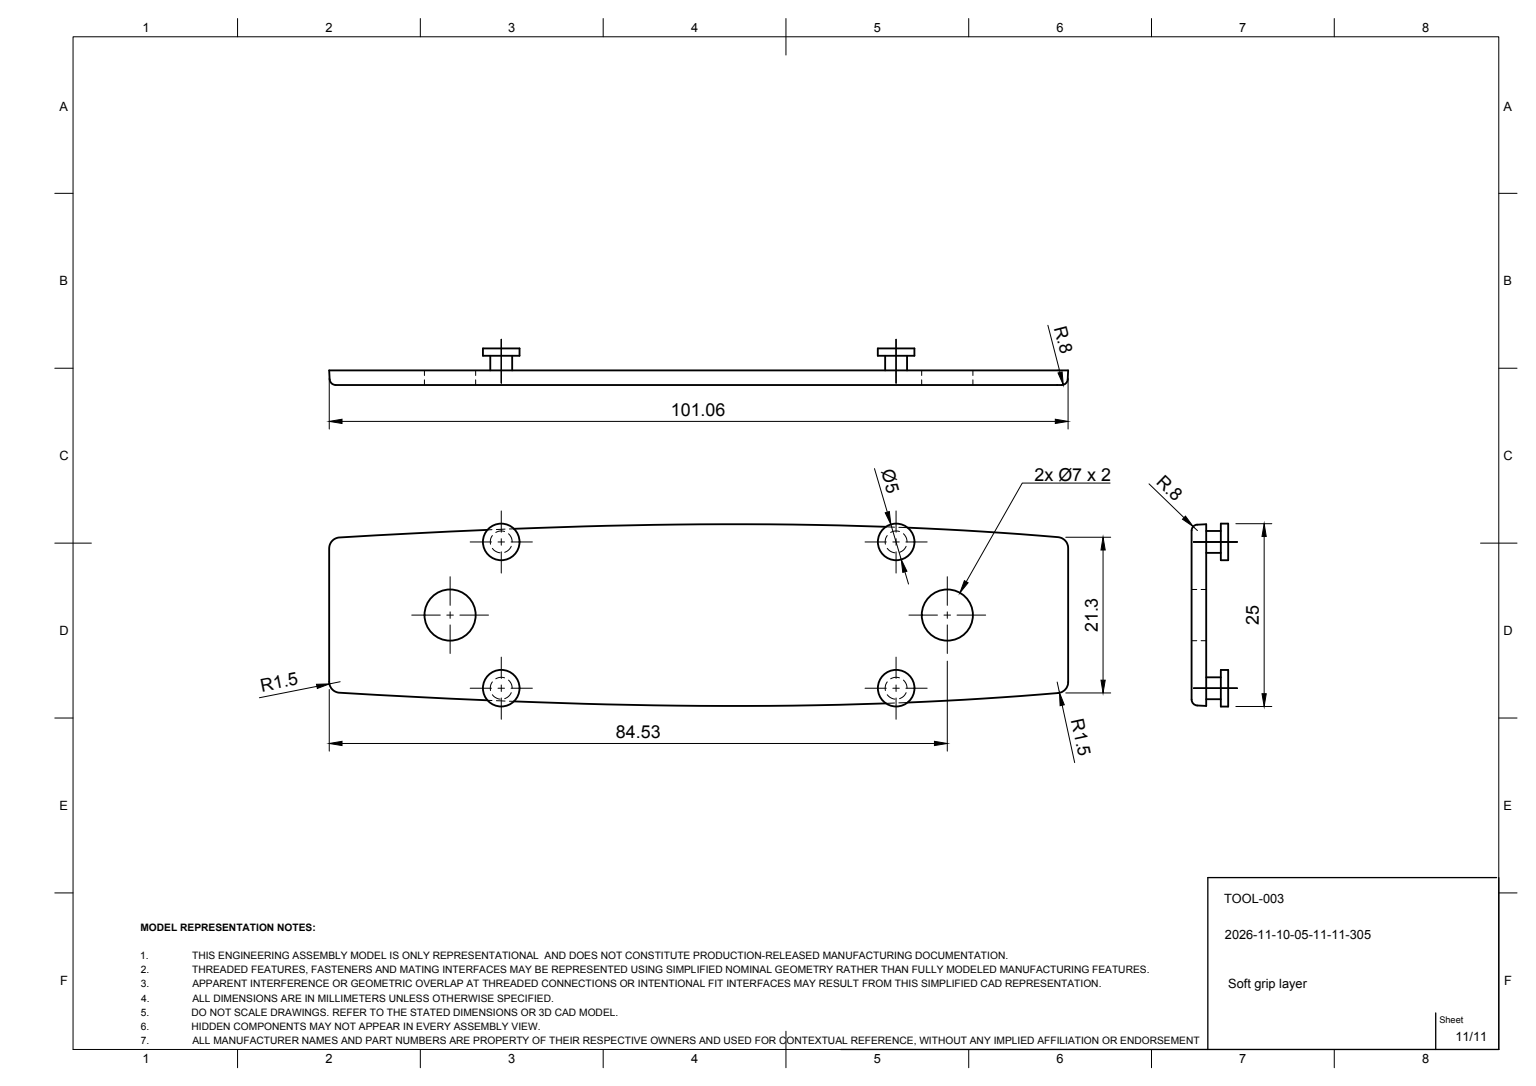
ISO-10303-21;
HEADER;
/* Generated by software containing ST-Developer
 * from STEP Tools, Inc. (www.steptools.com) 
 */

FILE_DESCRIPTION(
/* description */ (''),
/* implementation_level */ '2;1');

FILE_NAME(
/* name */ 'Soft grip layer.step',
/* time_stamp */ '2026-11-10T05:20:16-08:00',
/* author */ (''),
/* organization */ (''),
/* preprocessor_version */ 'ST-DEVELOPER v20.2',
/* originating_system */ 'Autodesk Translation Framework v15.17.0.0',
/* authorisation */ '');

FILE_SCHEMA (('AUTOMOTIVE_DESIGN { 1 0 10303 214 3 1 1 }'));
ENDSEC;

DATA;
#10=MECHANICAL_DESIGN_GEOMETRIC_PRESENTATION_REPRESENTATION('',(#120),#24809);
#100=SHAPE_REPRESENTATION_RELATIONSHIP('SRR','None',#24864,#110);
#110=ADVANCED_BREP_SHAPE_REPRESENTATION('',(#130),#24807);
#120=STYLED_ITEM('',(#24924),#130);
#130=MANIFOLD_SOLID_BREP('Body1',#9897);
#185=FACE_BOUND('',#2432,.T.);
#186=FACE_BOUND('',#2436,.T.);
#187=FACE_BOUND('',#2440,.T.);
#188=FACE_BOUND('',#2444,.T.);
#189=FACE_BOUND('',#2464,.T.);
#190=FACE_BOUND('',#2465,.T.);
#191=FACE_BOUND('',#2470,.T.);
#192=FACE_BOUND('',#2471,.T.);
#193=FACE_BOUND('',#2472,.T.);
#194=FACE_BOUND('',#2473,.T.);
#195=FACE_BOUND('',#2474,.T.);
#196=FACE_BOUND('',#2475,.T.);
#273=B_SPLINE_SURFACE_WITH_KNOTS('',3,3,((#24235,#24236,#24237,#24238,#24239),
(#24240,#24241,#24242,#24243,#24244),(#24245,#24246,#24247,#24248,#24249),
(#24250,#24251,#24252,#24253,#24254),(#24255,#24256,#24257,#24258,#24259)),
 .UNSPECIFIED.,.F.,.F.,.F.,(4,1,4),(4,1,4),(0.,0.571428571428571,1.),(0.,
0.0453052401185593,0.105712226943305),.UNSPECIFIED.);
#274=B_SPLINE_SURFACE_WITH_KNOTS('',3,3,((#24282,#24283,#24284,#24285,#24286),
(#24287,#24288,#24289,#24290,#24291),(#24292,#24293,#24294,#24295,#24296),
(#24297,#24298,#24299,#24300,#24301),(#24302,#24303,#24304,#24305,#24306)),
 .UNSPECIFIED.,.F.,.F.,.F.,(4,1,4),(4,1,4),(0.,0.571428571428571,1.),(0.,
0.0453052401439183,0.105712227002476),.UNSPECIFIED.);
#275=B_SPLINE_SURFACE_WITH_KNOTS('',3,3,((#24320,#24321,#24322,#24323,#24324),
(#24325,#24326,#24327,#24328,#24329),(#24330,#24331,#24332,#24333,#24334),
(#24335,#24336,#24337,#24338,#24339),(#24340,#24341,#24342,#24343,#24344)),
 .UNSPECIFIED.,.F.,.F.,.F.,(4,1,4),(4,1,4),(0.,0.571428571428571,1.),(0.,
4.20509945658767,9.8118987320379),.UNSPECIFIED.);
#276=B_SPLINE_SURFACE_WITH_KNOTS('',3,3,((#24358,#24359,#24360,#24361,#24362),
(#24363,#24364,#24365,#24366,#24367),(#24368,#24369,#24370,#24371,#24372),
(#24373,#24374,#24375,#24376,#24377),(#24378,#24379,#24380,#24381,#24382)),
 .UNSPECIFIED.,.F.,.F.,.F.,(4,1,4),(4,1,4),(0.,0.571428571428571,1.),(0.,
0.0444882141544403,0.103805833027027),.UNSPECIFIED.);
#277=B_SPLINE_SURFACE_WITH_KNOTS('',3,3,((#24402,#24403,#24404,#24405,#24406),
(#24407,#24408,#24409,#24410,#24411),(#24412,#24413,#24414,#24415,#24416),
(#24417,#24418,#24419,#24420,#24421),(#24422,#24423,#24424,#24425,#24426)),
 .UNSPECIFIED.,.F.,.F.,.F.,(4,1,4),(4,1,4),(0.,0.571428571428571,1.),(2.06005858395869E-18,
0.0444882141931362,0.103805833117318),.UNSPECIFIED.);
#278=B_SPLINE_SURFACE_WITH_KNOTS('',3,3,((#24440,#24441,#24442,#24443,#24444),
(#24445,#24446,#24447,#24448,#24449),(#24450,#24451,#24452,#24453,#24454),
(#24455,#24456,#24457,#24458,#24459),(#24460,#24461,#24462,#24463,#24464)),
 .UNSPECIFIED.,.F.,.F.,.F.,(4,1,4),(4,1,4),(0.,0.571428571428571,1.),(0.,
4.20509909783593,9.81189789495051),.UNSPECIFIED.);
#279=B_SPLINE_SURFACE_WITH_KNOTS('',3,3,((#24487,#24488,#24489,#24490),
(#24491,#24492,#24493,#24494),(#24495,#24496,#24497,#24498),(#24499,#24500,
#24501,#24502),(#24503,#24504,#24505,#24506)),.UNSPECIFIED.,.F.,.F.,.F.,
(4,1,4),(4,4),(0.,0.571428571428571,1.),(-0.00268702576369722,0.125151053668407),
 .UNSPECIFIED.);
#280=B_SPLINE_SURFACE_WITH_KNOTS('',3,3,((#24540,#24541,#24542,#24543),
(#24544,#24545,#24546,#24547),(#24548,#24549,#24550,#24551),(#24552,#24553,
#24554,#24555)),.UNSPECIFIED.,.F.,.F.,.F.,(4,4),(4,4),(0.0135518988075539,
0.986045335056424),(0.,0.622596671418298),.UNSPECIFIED.);
#281=B_SPLINE_SURFACE_WITH_KNOTS('',3,3,((#24565,#24566,#24567,#24568),
(#24569,#24570,#24571,#24572),(#24573,#24574,#24575,#24576),(#24577,#24578,
#24579,#24580),(#24581,#24582,#24583,#24584)),.UNSPECIFIED.,.F.,.F.,.F.,
(4,1,4),(4,4),(0.,0.571428571428571,1.),(-0.00281084541253883,0.124959300034279),
 .UNSPECIFIED.);
#282=B_SPLINE_SURFACE_WITH_KNOTS('',3,3,((#24626,#24627,#24628,#24629),
(#24630,#24631,#24632,#24633),(#24634,#24635,#24636,#24637),(#24638,#24639,
#24640,#24641),(#24642,#24643,#24644,#24645)),.UNSPECIFIED.,.F.,.F.,.F.,
(4,1,4),(4,4),(0.,0.571428571428571,1.),(-0.00261432509268751,0.125151053668407),
 .UNSPECIFIED.);
#283=B_SPLINE_SURFACE_WITH_KNOTS('',3,3,((#24679,#24680,#24681,#24682),
(#24683,#24684,#24685,#24686),(#24687,#24688,#24689,#24690),(#24691,#24692,
#24693,#24694),(#24695,#24696,#24697,#24698)),.UNSPECIFIED.,.F.,.F.,.F.,
(4,1,4),(4,4),(0.,0.571428571428571,1.),(-0.00286362952972032,0.124959300034279),
 .UNSPECIFIED.);
#284=B_SPLINE_SURFACE_WITH_KNOTS('',3,3,((#24737,#24738,#24739,#24740),
(#24741,#24742,#24743,#24744),(#24745,#24746,#24747,#24748),(#24749,#24750,
#24751,#24752)),.UNSPECIFIED.,.F.,.F.,.F.,(4,4),(4,4),(0.0139546649435754,
0.986448101192446),(0.,0.622596671418299),.UNSPECIFIED.);
#973=B_SPLINE_CURVE_WITH_KNOTS('',3,(#24264,#24265,#24266,#24267,#24268),
 .UNSPECIFIED.,.F.,.F.,(4,1,4),(-0.105712226943305,-0.0453052401185593,
0.),.UNSPECIFIED.);
#974=B_SPLINE_CURVE_WITH_KNOTS('',3,(#24271,#24272,#24273,#24274,#24275),
 .UNSPECIFIED.,.F.,.F.,(4,1,4),(0.,0.0453052401185593,0.105712226943305),
 .UNSPECIFIED.);
#975=B_SPLINE_CURVE_WITH_KNOTS('',3,(#24310,#24311,#24312,#24313,#24314),
 .UNSPECIFIED.,.F.,.F.,(4,1,4),(-0.105712227002476,-0.0453052401439183,
0.),.UNSPECIFIED.);
#976=B_SPLINE_CURVE_WITH_KNOTS('',3,(#24315,#24316,#24317,#24318,#24319),
 .UNSPECIFIED.,.F.,.F.,(4,1,4),(0.,0.0453052401439183,0.105712227002476),
 .UNSPECIFIED.);
#977=B_SPLINE_CURVE_WITH_KNOTS('',3,(#24348,#24349,#24350,#24351,#24352),
 .UNSPECIFIED.,.F.,.F.,(4,1,4),(-9.8118987320379,-4.20509945658767,0.),
 .UNSPECIFIED.);
#978=B_SPLINE_CURVE_WITH_KNOTS('',3,(#24353,#24354,#24355,#24356,#24357),
 .UNSPECIFIED.,.F.,.F.,(4,1,4),(0.,4.20509945658767,9.8118987320379),
 .UNSPECIFIED.);
#979=B_SPLINE_CURVE_WITH_KNOTS('',3,(#24386,#24387,#24388,#24389,#24390),
 .UNSPECIFIED.,.F.,.F.,(4,1,4),(-0.103805833027027,-0.0444882141544403,
0.),.UNSPECIFIED.);
#980=B_SPLINE_CURVE_WITH_KNOTS('',3,(#24391,#24392,#24393,#24394,#24395),
 .UNSPECIFIED.,.F.,.F.,(4,1,4),(0.,0.0444882141544403,0.103805833027027),
 .UNSPECIFIED.);
#981=B_SPLINE_CURVE_WITH_KNOTS('',3,(#24430,#24431,#24432,#24433,#24434),
 .UNSPECIFIED.,.F.,.F.,(4,1,4),(-0.103805833117318,-0.0444882141931362,
-2.06005858395869E-18),.UNSPECIFIED.);
#982=B_SPLINE_CURVE_WITH_KNOTS('',3,(#24435,#24436,#24437,#24438,#24439),
 .UNSPECIFIED.,.F.,.F.,(4,1,4),(2.06005858395869E-18,0.0444882141931362,
0.103805833117318),.UNSPECIFIED.);
#983=B_SPLINE_CURVE_WITH_KNOTS('',3,(#24465,#24466,#24467,#24468,#24469),
 .UNSPECIFIED.,.F.,.F.,(4,1,4),(-9.81189789495051,-4.20509909783593,0.),
 .UNSPECIFIED.);
#984=B_SPLINE_CURVE_WITH_KNOTS('',3,(#24470,#24471,#24472,#24473,#24474),
 .UNSPECIFIED.,.F.,.F.,(4,1,4),(0.,4.20509909783593,9.81189789495051),
 .UNSPECIFIED.);
#985=B_SPLINE_CURVE_WITH_KNOTS('',3,(#24477,#24478,#24479,#24480),
 .UNSPECIFIED.,.F.,.F.,(4,4),(0.00062434729305816,0.125151053668407),
 .UNSPECIFIED.);
#986=B_SPLINE_CURVE_WITH_KNOTS('',3,(#24483,#24484,#24485,#24486),
 .UNSPECIFIED.,.F.,.F.,(4,4),(-0.125151053668407,-0.000624347293058304),
 .UNSPECIFIED.);
#987=B_SPLINE_CURVE_WITH_KNOTS('',3,(#24508,#24509,#24510,#24511),
 .UNSPECIFIED.,.F.,.F.,(4,4),(-0.124859357077656,3.91613824701764E-16),
 .UNSPECIFIED.);
#988=B_SPLINE_CURVE_WITH_KNOTS('',3,(#24512,#24513,#24514,#24515,#24516,
#24517,#24518,#24519,#24520,#24521,#24522,#24523,#24524,#24525,#24526,#24527,
#24528,#24529,#24530,#24531,#24532,#24533,#24534,#24535,#24536,#24537,#24538,
#24539),.UNSPECIFIED.,.F.,.F.,(4,3,3,3,3,3,3,3,3,4),(0.,0.0322709922822142,
0.0586131010579366,0.0908535483049993,0.095660418056781,0.117090121226367,
0.14947943031994,0.17008966569926,0.202270498561131,0.223122165115773),
 .UNSPECIFIED.);
#989=B_SPLINE_CURVE_WITH_KNOTS('',3,(#24557,#24558,#24559,#24560),
 .UNSPECIFIED.,.F.,.F.,(4,4),(1.57426155444895E-16,0.124757292074316),
 .UNSPECIFIED.);
#990=B_SPLINE_CURVE_WITH_KNOTS('',3,(#24561,#24562,#24563,#24564),
 .UNSPECIFIED.,.F.,.F.,(4,4),(0.0135518988075539,0.986045335056425),
 .UNSPECIFIED.);
#991=B_SPLINE_CURVE_WITH_KNOTS('',3,(#24586,#24587,#24588,#24589),
 .UNSPECIFIED.,.F.,.F.,(4,4),(-0.124959300034279,-0.000432357919845506),
 .UNSPECIFIED.);
#992=B_SPLINE_CURVE_WITH_KNOTS('',3,(#24590,#24591,#24592,#24593,#24594,
#24595,#24596,#24597,#24598,#24599,#24600,#24601,#24602,#24603,#24604,#24605,
#24606,#24607,#24608,#24609,#24610,#24611,#24612,#24613,#24614,#24615,#24616,
#24617),.UNSPECIFIED.,.F.,.F.,(4,3,3,3,3,3,3,3,3,4),(0.,0.0322720371751271,
0.0586511315716134,0.0908889384397039,0.0974306796249642,0.117149930269381,
0.149553095257184,0.172178760978465,0.204364325027201,0.227238249760569),
 .UNSPECIFIED.);
#993=B_SPLINE_CURVE_WITH_KNOTS('',3,(#24621,#24622,#24623,#24624),
 .UNSPECIFIED.,.F.,.F.,(4,4),(0.000432357919845864,0.124959300034279),
 .UNSPECIFIED.);
#994=B_SPLINE_CURVE_WITH_KNOTS('',3,(#24647,#24648,#24649,#24650,#24651,
#24652,#24653,#24654,#24655,#24656,#24657,#24658,#24659,#24660,#24661,#24662,
#24663,#24664,#24665,#24666,#24667,#24668,#24669,#24670,#24671,#24672,#24673,
#24674),.UNSPECIFIED.,.F.,.F.,(4,3,3,3,3,3,3,3,3,4),(0.,0.0322770007607458,
0.0586509099358757,0.0908890592373506,0.0956758252683957,0.117149647541228,
0.149540928065794,0.17012301918783,0.202296660223156,0.2231241621482),
 .UNSPECIFIED.);
#995=B_SPLINE_CURVE_WITH_KNOTS('',3,(#24675,#24676,#24677,#24678),
 .UNSPECIFIED.,.F.,.F.,(4,4),(1.94722710178397E-16,0.124859357077656),
 .UNSPECIFIED.);
#996=B_SPLINE_CURVE_WITH_KNOTS('',3,(#24700,#24701,#24702,#24703),
 .UNSPECIFIED.,.F.,.F.,(4,4),(-0.124757292074297,-2.43294967505747E-16),
 .UNSPECIFIED.);
#997=B_SPLINE_CURVE_WITH_KNOTS('',3,(#24704,#24705,#24706,#24707,#24708,
#24709,#24710,#24711,#24712,#24713,#24714,#24715,#24716,#24717,#24718,#24719,
#24720,#24721,#24722,#24723,#24724,#24725,#24726,#24727,#24728,#24729,#24730,
#24731),.UNSPECIFIED.,.F.,.F.,(4,3,3,3,3,3,3,3,3,4),(0.,0.0322677829554273,
0.0586251784806003,0.0908644978360146,0.097419835848357,0.117108565494702,
0.149510109206484,0.172155480916619,0.204345933772221,0.227236831322489),
 .UNSPECIFIED.);
#998=B_SPLINE_CURVE_WITH_KNOTS('',3,(#24733,#24734,#24735,#24736),
 .UNSPECIFIED.,.F.,.F.,(4,4),(0.0139546649435756,0.986448101192446),
 .UNSPECIFIED.);
#1296=PLANE('',#10602);
#1297=PLANE('',#10607);
#1298=PLANE('',#10608);
#1299=PLANE('',#10613);
#1300=PLANE('',#10614);
#1301=PLANE('',#10619);
#1302=PLANE('',#10620);
#1303=PLANE('',#10625);
#1304=PLANE('',#10644);
#1305=PLANE('',#10645);
#1306=PLANE('',#10646);
#1307=PLANE('',#10647);
#1823=FACE_OUTER_BOUND('',#2429,.T.);
#1824=FACE_OUTER_BOUND('',#2430,.T.);
#1825=FACE_OUTER_BOUND('',#2431,.T.);
#1826=FACE_OUTER_BOUND('',#2433,.T.);
#1827=FACE_OUTER_BOUND('',#2434,.T.);
#1828=FACE_OUTER_BOUND('',#2435,.T.);
#1829=FACE_OUTER_BOUND('',#2437,.T.);
#1830=FACE_OUTER_BOUND('',#2438,.T.);
#1831=FACE_OUTER_BOUND('',#2439,.T.);
#1832=FACE_OUTER_BOUND('',#2441,.T.);
#1833=FACE_OUTER_BOUND('',#2442,.T.);
#1834=FACE_OUTER_BOUND('',#2443,.T.);
#1835=FACE_OUTER_BOUND('',#2445,.T.);
#1836=FACE_OUTER_BOUND('',#2446,.T.);
#1837=FACE_OUTER_BOUND('',#2447,.T.);
#1838=FACE_OUTER_BOUND('',#2448,.T.);
#1839=FACE_OUTER_BOUND('',#2449,.T.);
#1840=FACE_OUTER_BOUND('',#2450,.T.);
#1841=FACE_OUTER_BOUND('',#2451,.T.);
#1842=FACE_OUTER_BOUND('',#2452,.T.);
#1843=FACE_OUTER_BOUND('',#2453,.T.);
#1844=FACE_OUTER_BOUND('',#2454,.T.);
#1845=FACE_OUTER_BOUND('',#2455,.T.);
#1846=FACE_OUTER_BOUND('',#2456,.T.);
#1847=FACE_OUTER_BOUND('',#2457,.T.);
#1848=FACE_OUTER_BOUND('',#2458,.T.);
#1849=FACE_OUTER_BOUND('',#2459,.T.);
#1850=FACE_OUTER_BOUND('',#2460,.T.);
#1851=FACE_OUTER_BOUND('',#2461,.T.);
#1852=FACE_OUTER_BOUND('',#2462,.T.);
#1853=FACE_OUTER_BOUND('',#2463,.T.);
#1854=FACE_OUTER_BOUND('',#2466,.T.);
#1855=FACE_OUTER_BOUND('',#2467,.T.);
#1856=FACE_OUTER_BOUND('',#2468,.T.);
#1857=FACE_OUTER_BOUND('',#2469,.T.);
#1858=FACE_OUTER_BOUND('',#2476,.T.);
#2429=EDGE_LOOP('',(#9045,#9046,#9047,#9048));
#2430=EDGE_LOOP('',(#9049,#9050,#9051,#9052));
#2431=EDGE_LOOP('',(#9053));
#2432=EDGE_LOOP('',(#9054));
#2433=EDGE_LOOP('',(#9055,#9056,#9057,#9058));
#2434=EDGE_LOOP('',(#9059));
#2435=EDGE_LOOP('',(#9060));
#2436=EDGE_LOOP('',(#9061));
#2437=EDGE_LOOP('',(#9062,#9063,#9064,#9065));
#2438=EDGE_LOOP('',(#9066));
#2439=EDGE_LOOP('',(#9067));
#2440=EDGE_LOOP('',(#9068));
#2441=EDGE_LOOP('',(#9069,#9070,#9071,#9072));
#2442=EDGE_LOOP('',(#9073));
#2443=EDGE_LOOP('',(#9074));
#2444=EDGE_LOOP('',(#9075));
#2445=EDGE_LOOP('',(#9076,#9077,#9078,#9079));
#2446=EDGE_LOOP('',(#9080));
#2447=EDGE_LOOP('',(#9081,#9082,#9083,#9084));
#2448=EDGE_LOOP('',(#9085,#9086,#9087,#9088));
#2449=EDGE_LOOP('',(#9089,#9090,#9091,#9092));
#2450=EDGE_LOOP('',(#9093,#9094,#9095,#9096));
#2451=EDGE_LOOP('',(#9097,#9098,#9099,#9100));
#2452=EDGE_LOOP('',(#9101,#9102,#9103,#9104));
#2453=EDGE_LOOP('',(#9105,#9106,#9107,#9108));
#2454=EDGE_LOOP('',(#9109,#9110,#9111,#9112));
#2455=EDGE_LOOP('',(#9113,#9114,#9115,#9116));
#2456=EDGE_LOOP('',(#9117,#9118,#9119,#9120));
#2457=EDGE_LOOP('',(#9121,#9122,#9123,#9124));
#2458=EDGE_LOOP('',(#9125,#9126,#9127,#9128));
#2459=EDGE_LOOP('',(#9129,#9130,#9131,#9132));
#2460=EDGE_LOOP('',(#9133,#9134,#9135,#9136));
#2461=EDGE_LOOP('',(#9137,#9138,#9139,#9140));
#2462=EDGE_LOOP('',(#9141,#9142,#9143,#9144));
#2463=EDGE_LOOP('',(#9145,#9146,#9147,#9148,#9149,#9150,#9151,#9152));
#2464=EDGE_LOOP('',(#9153));
#2465=EDGE_LOOP('',(#9154));
#2466=EDGE_LOOP('',(#9155,#9156,#9157,#9158));
#2467=EDGE_LOOP('',(#9159,#9160,#9161,#9162));
#2468=EDGE_LOOP('',(#9163,#9164,#9165,#9166));
#2469=EDGE_LOOP('',(#9167,#9168,#9169,#9170,#9171,#9172,#9173,#9174));
#2470=EDGE_LOOP('',(#9175));
#2471=EDGE_LOOP('',(#9176));
#2472=EDGE_LOOP('',(#9177));
#2473=EDGE_LOOP('',(#9178));
#2474=EDGE_LOOP('',(#9179));
#2475=EDGE_LOOP('',(#9180));
#2476=EDGE_LOOP('',(#9181,#9182,#9183,#9184));
#3053=LINE('',#24171,#3641);
#3054=LINE('',#24177,#3642);
#3055=LINE('',#24187,#3643);
#3056=LINE('',#24197,#3644);
#3057=LINE('',#24207,#3645);
#3058=LINE('',#24217,#3646);
#3059=LINE('',#24221,#3647);
#3060=LINE('',#24225,#3648);
#3061=LINE('',#24229,#3649);
#3062=LINE('',#24233,#3650);
#3063=LINE('',#24280,#3651);
#3064=LINE('',#24281,#3652);
#3065=LINE('',#24400,#3653);
#3066=LINE('',#24401,#3654);
#3067=LINE('',#24482,#3655);
#3068=LINE('',#24625,#3656);
#3641=VECTOR('',#12419,0.35);
#3642=VECTOR('',#12426,0.35);
#3643=VECTOR('',#12439,0.25);
#3644=VECTOR('',#12452,0.25);
#3645=VECTOR('',#12465,0.25);
#3646=VECTOR('',#12478,0.25);
#3647=VECTOR('',#12483,0.15);
#3648=VECTOR('',#12488,0.15);
#3649=VECTOR('',#12493,0.15);
#3650=VECTOR('',#12498,0.15);
#3651=VECTOR('',#12509,1.);
#3652=VECTOR('',#12510,1.);
#3653=VECTOR('',#12521,1.);
#3654=VECTOR('',#12522,1.);
#3655=VECTOR('',#12527,1.);
#3656=VECTOR('',#12532,1.);
#3795=CIRCLE('',#10597,0.35);
#3796=CIRCLE('',#10598,0.35);
#3797=CIRCLE('',#10600,0.35);
#3798=CIRCLE('',#10601,0.35);
#3799=CIRCLE('',#10603,0.25);
#3800=CIRCLE('',#10604,0.15);
#3801=CIRCLE('',#10606,0.25);
#3802=CIRCLE('',#10609,0.25);
#3803=CIRCLE('',#10610,0.15);
#3804=CIRCLE('',#10612,0.25);
#3805=CIRCLE('',#10615,0.25);
#3806=CIRCLE('',#10616,0.15);
#3807=CIRCLE('',#10618,0.25);
#3808=CIRCLE('',#10621,0.25);
#3809=CIRCLE('',#10622,0.15);
#3810=CIRCLE('',#10624,0.25);
#3811=CIRCLE('',#10627,0.15);
#3812=CIRCLE('',#10629,0.15);
#3813=CIRCLE('',#10631,0.15);
#3814=CIRCLE('',#10633,0.15);
#3815=CIRCLE('',#10634,0.0800000000000001);
#3816=CIRCLE('',#10635,0.0799999999999999);
#3817=CIRCLE('',#10637,0.0800000000000001);
#3818=CIRCLE('',#10638,0.0800000000000001);
#3819=CIRCLE('',#10639,0.0800000000000001);
#3820=CIRCLE('',#10640,0.0800000000000001);
#3821=CIRCLE('',#10642,0.0800000000000001);
#3822=CIRCLE('',#10643,0.0800000000000001);
#4739=VERTEX_POINT('',#24168);
#4740=VERTEX_POINT('',#24170);
#4741=VERTEX_POINT('',#24174);
#4742=VERTEX_POINT('',#24176);
#4743=VERTEX_POINT('',#24180);
#4744=VERTEX_POINT('',#24182);
#4745=VERTEX_POINT('',#24185);
#4746=VERTEX_POINT('',#24190);
#4747=VERTEX_POINT('',#24192);
#4748=VERTEX_POINT('',#24195);
#4749=VERTEX_POINT('',#24200);
#4750=VERTEX_POINT('',#24202);
#4751=VERTEX_POINT('',#24205);
#4752=VERTEX_POINT('',#24210);
#4753=VERTEX_POINT('',#24212);
#4754=VERTEX_POINT('',#24215);
#4755=VERTEX_POINT('',#24220);
#4756=VERTEX_POINT('',#24224);
#4757=VERTEX_POINT('',#24228);
#4758=VERTEX_POINT('',#24232);
#4759=VERTEX_POINT('',#24260);
#4760=VERTEX_POINT('',#24261);
#4761=VERTEX_POINT('',#24263);
#4762=VERTEX_POINT('',#24269);
#4763=VERTEX_POINT('',#24277);
#4764=VERTEX_POINT('',#24278);
#4765=VERTEX_POINT('',#24307);
#4766=VERTEX_POINT('',#24308);
#4767=VERTEX_POINT('',#24345);
#4768=VERTEX_POINT('',#24346);
#4769=VERTEX_POINT('',#24383);
#4770=VERTEX_POINT('',#24384);
#4771=VERTEX_POINT('',#24397);
#4772=VERTEX_POINT('',#24398);
#4773=VERTEX_POINT('',#24427);
#4774=VERTEX_POINT('',#24428);
#4775=VERTEX_POINT('',#24476);
#4776=VERTEX_POINT('',#24481);
#4777=VERTEX_POINT('',#24507);
#4778=VERTEX_POINT('',#24556);
#4779=VERTEX_POINT('',#24585);
#4780=VERTEX_POINT('',#24620);
#4781=VERTEX_POINT('',#24646);
#4782=VERTEX_POINT('',#24699);
#6181=EDGE_CURVE('',#4739,#4739,#3795,.T.);
#6182=EDGE_CURVE('',#4739,#4740,#3053,.T.);
#6183=EDGE_CURVE('',#4740,#4740,#3796,.T.);
#6184=EDGE_CURVE('',#4741,#4741,#3797,.T.);
#6185=EDGE_CURVE('',#4741,#4742,#3054,.T.);
#6186=EDGE_CURVE('',#4742,#4742,#3798,.T.);
#6187=EDGE_CURVE('',#4743,#4743,#3799,.T.);
#6188=EDGE_CURVE('',#4744,#4744,#3800,.T.);
#6189=EDGE_CURVE('',#4745,#4745,#3801,.T.);
#6190=EDGE_CURVE('',#4745,#4743,#3055,.T.);
#6191=EDGE_CURVE('',#4746,#4746,#3802,.T.);
#6192=EDGE_CURVE('',#4747,#4747,#3803,.T.);
#6193=EDGE_CURVE('',#4748,#4748,#3804,.T.);
#6194=EDGE_CURVE('',#4748,#4746,#3056,.T.);
#6195=EDGE_CURVE('',#4749,#4749,#3805,.T.);
#6196=EDGE_CURVE('',#4750,#4750,#3806,.T.);
#6197=EDGE_CURVE('',#4751,#4751,#3807,.T.);
#6198=EDGE_CURVE('',#4751,#4749,#3057,.T.);
#6199=EDGE_CURVE('',#4752,#4752,#3808,.T.);
#6200=EDGE_CURVE('',#4753,#4753,#3809,.T.);
#6201=EDGE_CURVE('',#4754,#4754,#3810,.T.);
#6202=EDGE_CURVE('',#4754,#4752,#3058,.T.);
#6203=EDGE_CURVE('',#4744,#4755,#3059,.T.);
#6204=EDGE_CURVE('',#4755,#4755,#3811,.T.);
#6205=EDGE_CURVE('',#4747,#4756,#3060,.T.);
#6206=EDGE_CURVE('',#4756,#4756,#3812,.T.);
#6207=EDGE_CURVE('',#4750,#4757,#3061,.T.);
#6208=EDGE_CURVE('',#4757,#4757,#3813,.T.);
#6209=EDGE_CURVE('',#4753,#4758,#3062,.T.);
#6210=EDGE_CURVE('',#4758,#4758,#3814,.T.);
#6211=EDGE_CURVE('',#4759,#4760,#3815,.T.);
#6212=EDGE_CURVE('',#4760,#4761,#973,.T.);
#6213=EDGE_CURVE('',#4761,#4762,#3816,.T.);
#6214=EDGE_CURVE('',#4762,#4759,#974,.T.);
#6215=EDGE_CURVE('',#4763,#4764,#3817,.T.);
#6216=EDGE_CURVE('',#4764,#4760,#3063,.T.);
#6217=EDGE_CURVE('',#4759,#4763,#3064,.T.);
#6218=EDGE_CURVE('',#4765,#4766,#3818,.T.);
#6219=EDGE_CURVE('',#4766,#4764,#975,.T.);
#6220=EDGE_CURVE('',#4763,#4765,#976,.T.);
#6221=EDGE_CURVE('',#4767,#4768,#3819,.T.);
#6222=EDGE_CURVE('',#4768,#4766,#977,.T.);
#6223=EDGE_CURVE('',#4765,#4767,#978,.T.);
#6224=EDGE_CURVE('',#4769,#4770,#3820,.T.);
#6225=EDGE_CURVE('',#4770,#4768,#979,.T.);
#6226=EDGE_CURVE('',#4767,#4769,#980,.T.);
#6227=EDGE_CURVE('',#4771,#4772,#3821,.T.);
#6228=EDGE_CURVE('',#4772,#4770,#3065,.T.);
#6229=EDGE_CURVE('',#4769,#4771,#3066,.T.);
#6230=EDGE_CURVE('',#4773,#4774,#3822,.T.);
#6231=EDGE_CURVE('',#4774,#4772,#981,.T.);
#6232=EDGE_CURVE('',#4771,#4773,#982,.T.);
#6233=EDGE_CURVE('',#4761,#4774,#983,.T.);
#6234=EDGE_CURVE('',#4773,#4762,#984,.T.);
#6235=EDGE_CURVE('',#4775,#4772,#985,.T.);
#6236=EDGE_CURVE('',#4776,#4775,#3067,.T.);
#6237=EDGE_CURVE('',#4770,#4776,#986,.T.);
#6238=EDGE_CURVE('',#4774,#4777,#987,.T.);
#6239=EDGE_CURVE('',#4777,#4775,#988,.T.);
#6240=EDGE_CURVE('',#4778,#4761,#989,.T.);
#6241=EDGE_CURVE('',#4777,#4778,#990,.T.);
#6242=EDGE_CURVE('',#4760,#4779,#991,.T.);
#6243=EDGE_CURVE('',#4779,#4778,#992,.T.);
#6244=EDGE_CURVE('',#4780,#4764,#993,.T.);
#6245=EDGE_CURVE('',#4779,#4780,#3068,.T.);
#6246=EDGE_CURVE('',#4776,#4781,#994,.T.);
#6247=EDGE_CURVE('',#4781,#4768,#995,.T.);
#6248=EDGE_CURVE('',#4766,#4782,#996,.T.);
#6249=EDGE_CURVE('',#4782,#4780,#997,.T.);
#6250=EDGE_CURVE('',#4782,#4781,#998,.T.);
#9045=ORIENTED_EDGE('',*,*,#6181,.F.);
#9046=ORIENTED_EDGE('',*,*,#6182,.T.);
#9047=ORIENTED_EDGE('',*,*,#6183,.F.);
#9048=ORIENTED_EDGE('',*,*,#6182,.F.);
#9049=ORIENTED_EDGE('',*,*,#6184,.F.);
#9050=ORIENTED_EDGE('',*,*,#6185,.T.);
#9051=ORIENTED_EDGE('',*,*,#6186,.F.);
#9052=ORIENTED_EDGE('',*,*,#6185,.F.);
#9053=ORIENTED_EDGE('',*,*,#6187,.T.);
#9054=ORIENTED_EDGE('',*,*,#6188,.T.);
#9055=ORIENTED_EDGE('',*,*,#6189,.F.);
#9056=ORIENTED_EDGE('',*,*,#6190,.T.);
#9057=ORIENTED_EDGE('',*,*,#6187,.F.);
#9058=ORIENTED_EDGE('',*,*,#6190,.F.);
#9059=ORIENTED_EDGE('',*,*,#6189,.T.);
#9060=ORIENTED_EDGE('',*,*,#6191,.T.);
#9061=ORIENTED_EDGE('',*,*,#6192,.T.);
#9062=ORIENTED_EDGE('',*,*,#6193,.F.);
#9063=ORIENTED_EDGE('',*,*,#6194,.T.);
#9064=ORIENTED_EDGE('',*,*,#6191,.F.);
#9065=ORIENTED_EDGE('',*,*,#6194,.F.);
#9066=ORIENTED_EDGE('',*,*,#6193,.T.);
#9067=ORIENTED_EDGE('',*,*,#6195,.T.);
#9068=ORIENTED_EDGE('',*,*,#6196,.T.);
#9069=ORIENTED_EDGE('',*,*,#6197,.F.);
#9070=ORIENTED_EDGE('',*,*,#6198,.T.);
#9071=ORIENTED_EDGE('',*,*,#6195,.F.);
#9072=ORIENTED_EDGE('',*,*,#6198,.F.);
#9073=ORIENTED_EDGE('',*,*,#6197,.T.);
#9074=ORIENTED_EDGE('',*,*,#6199,.T.);
#9075=ORIENTED_EDGE('',*,*,#6200,.T.);
#9076=ORIENTED_EDGE('',*,*,#6201,.F.);
#9077=ORIENTED_EDGE('',*,*,#6202,.T.);
#9078=ORIENTED_EDGE('',*,*,#6199,.F.);
#9079=ORIENTED_EDGE('',*,*,#6202,.F.);
#9080=ORIENTED_EDGE('',*,*,#6201,.T.);
#9081=ORIENTED_EDGE('',*,*,#6188,.F.);
#9082=ORIENTED_EDGE('',*,*,#6203,.T.);
#9083=ORIENTED_EDGE('',*,*,#6204,.F.);
#9084=ORIENTED_EDGE('',*,*,#6203,.F.);
#9085=ORIENTED_EDGE('',*,*,#6192,.F.);
#9086=ORIENTED_EDGE('',*,*,#6205,.T.);
#9087=ORIENTED_EDGE('',*,*,#6206,.F.);
#9088=ORIENTED_EDGE('',*,*,#6205,.F.);
#9089=ORIENTED_EDGE('',*,*,#6196,.F.);
#9090=ORIENTED_EDGE('',*,*,#6207,.T.);
#9091=ORIENTED_EDGE('',*,*,#6208,.F.);
#9092=ORIENTED_EDGE('',*,*,#6207,.F.);
#9093=ORIENTED_EDGE('',*,*,#6200,.F.);
#9094=ORIENTED_EDGE('',*,*,#6209,.T.);
#9095=ORIENTED_EDGE('',*,*,#6210,.F.);
#9096=ORIENTED_EDGE('',*,*,#6209,.F.);
#9097=ORIENTED_EDGE('',*,*,#6211,.T.);
#9098=ORIENTED_EDGE('',*,*,#6212,.T.);
#9099=ORIENTED_EDGE('',*,*,#6213,.T.);
#9100=ORIENTED_EDGE('',*,*,#6214,.T.);
#9101=ORIENTED_EDGE('',*,*,#6215,.T.);
#9102=ORIENTED_EDGE('',*,*,#6216,.T.);
#9103=ORIENTED_EDGE('',*,*,#6211,.F.);
#9104=ORIENTED_EDGE('',*,*,#6217,.T.);
#9105=ORIENTED_EDGE('',*,*,#6218,.T.);
#9106=ORIENTED_EDGE('',*,*,#6219,.T.);
#9107=ORIENTED_EDGE('',*,*,#6215,.F.);
#9108=ORIENTED_EDGE('',*,*,#6220,.T.);
#9109=ORIENTED_EDGE('',*,*,#6221,.T.);
#9110=ORIENTED_EDGE('',*,*,#6222,.T.);
#9111=ORIENTED_EDGE('',*,*,#6218,.F.);
#9112=ORIENTED_EDGE('',*,*,#6223,.T.);
#9113=ORIENTED_EDGE('',*,*,#6224,.T.);
#9114=ORIENTED_EDGE('',*,*,#6225,.T.);
#9115=ORIENTED_EDGE('',*,*,#6221,.F.);
#9116=ORIENTED_EDGE('',*,*,#6226,.T.);
#9117=ORIENTED_EDGE('',*,*,#6227,.T.);
#9118=ORIENTED_EDGE('',*,*,#6228,.T.);
#9119=ORIENTED_EDGE('',*,*,#6224,.F.);
#9120=ORIENTED_EDGE('',*,*,#6229,.T.);
#9121=ORIENTED_EDGE('',*,*,#6230,.T.);
#9122=ORIENTED_EDGE('',*,*,#6231,.T.);
#9123=ORIENTED_EDGE('',*,*,#6227,.F.);
#9124=ORIENTED_EDGE('',*,*,#6232,.T.);
#9125=ORIENTED_EDGE('',*,*,#6213,.F.);
#9126=ORIENTED_EDGE('',*,*,#6233,.T.);
#9127=ORIENTED_EDGE('',*,*,#6230,.F.);
#9128=ORIENTED_EDGE('',*,*,#6234,.T.);
#9129=ORIENTED_EDGE('',*,*,#6228,.F.);
#9130=ORIENTED_EDGE('',*,*,#6235,.F.);
#9131=ORIENTED_EDGE('',*,*,#6236,.F.);
#9132=ORIENTED_EDGE('',*,*,#6237,.F.);
#9133=ORIENTED_EDGE('',*,*,#6231,.F.);
#9134=ORIENTED_EDGE('',*,*,#6238,.T.);
#9135=ORIENTED_EDGE('',*,*,#6239,.T.);
#9136=ORIENTED_EDGE('',*,*,#6235,.T.);
#9137=ORIENTED_EDGE('',*,*,#6233,.F.);
#9138=ORIENTED_EDGE('',*,*,#6240,.F.);
#9139=ORIENTED_EDGE('',*,*,#6241,.F.);
#9140=ORIENTED_EDGE('',*,*,#6238,.F.);
#9141=ORIENTED_EDGE('',*,*,#6212,.F.);
#9142=ORIENTED_EDGE('',*,*,#6242,.T.);
#9143=ORIENTED_EDGE('',*,*,#6243,.T.);
#9144=ORIENTED_EDGE('',*,*,#6240,.T.);
#9145=ORIENTED_EDGE('',*,*,#6214,.F.);
#9146=ORIENTED_EDGE('',*,*,#6234,.F.);
#9147=ORIENTED_EDGE('',*,*,#6232,.F.);
#9148=ORIENTED_EDGE('',*,*,#6229,.F.);
#9149=ORIENTED_EDGE('',*,*,#6226,.F.);
#9150=ORIENTED_EDGE('',*,*,#6223,.F.);
#9151=ORIENTED_EDGE('',*,*,#6220,.F.);
#9152=ORIENTED_EDGE('',*,*,#6217,.F.);
#9153=ORIENTED_EDGE('',*,*,#6181,.T.);
#9154=ORIENTED_EDGE('',*,*,#6184,.T.);
#9155=ORIENTED_EDGE('',*,*,#6216,.F.);
#9156=ORIENTED_EDGE('',*,*,#6244,.F.);
#9157=ORIENTED_EDGE('',*,*,#6245,.F.);
#9158=ORIENTED_EDGE('',*,*,#6242,.F.);
#9159=ORIENTED_EDGE('',*,*,#6225,.F.);
#9160=ORIENTED_EDGE('',*,*,#6237,.T.);
#9161=ORIENTED_EDGE('',*,*,#6246,.T.);
#9162=ORIENTED_EDGE('',*,*,#6247,.T.);
#9163=ORIENTED_EDGE('',*,*,#6219,.F.);
#9164=ORIENTED_EDGE('',*,*,#6248,.T.);
#9165=ORIENTED_EDGE('',*,*,#6249,.T.);
#9166=ORIENTED_EDGE('',*,*,#6244,.T.);
#9167=ORIENTED_EDGE('',*,*,#6243,.F.);
#9168=ORIENTED_EDGE('',*,*,#6245,.T.);
#9169=ORIENTED_EDGE('',*,*,#6249,.F.);
#9170=ORIENTED_EDGE('',*,*,#6250,.T.);
#9171=ORIENTED_EDGE('',*,*,#6246,.F.);
#9172=ORIENTED_EDGE('',*,*,#6236,.T.);
#9173=ORIENTED_EDGE('',*,*,#6239,.F.);
#9174=ORIENTED_EDGE('',*,*,#6241,.T.);
#9175=ORIENTED_EDGE('',*,*,#6183,.T.);
#9176=ORIENTED_EDGE('',*,*,#6186,.T.);
#9177=ORIENTED_EDGE('',*,*,#6204,.T.);
#9178=ORIENTED_EDGE('',*,*,#6206,.T.);
#9179=ORIENTED_EDGE('',*,*,#6208,.T.);
#9180=ORIENTED_EDGE('',*,*,#6210,.T.);
#9181=ORIENTED_EDGE('',*,*,#6222,.F.);
#9182=ORIENTED_EDGE('',*,*,#6247,.F.);
#9183=ORIENTED_EDGE('',*,*,#6250,.F.);
#9184=ORIENTED_EDGE('',*,*,#6248,.F.);
#9322=CYLINDRICAL_SURFACE('',#10596,0.35);
#9323=CYLINDRICAL_SURFACE('',#10599,0.35);
#9324=CYLINDRICAL_SURFACE('',#10605,0.25);
#9325=CYLINDRICAL_SURFACE('',#10611,0.25);
#9326=CYLINDRICAL_SURFACE('',#10617,0.25);
#9327=CYLINDRICAL_SURFACE('',#10623,0.25);
#9328=CYLINDRICAL_SURFACE('',#10626,0.15);
#9329=CYLINDRICAL_SURFACE('',#10628,0.15);
#9330=CYLINDRICAL_SURFACE('',#10630,0.15);
#9331=CYLINDRICAL_SURFACE('',#10632,0.15);
#9332=CYLINDRICAL_SURFACE('',#10636,0.08);
#9333=CYLINDRICAL_SURFACE('',#10641,0.08);
#9849=ADVANCED_FACE('',(#1823),#9322,.F.);
#9850=ADVANCED_FACE('',(#1824),#9323,.F.);
#9851=ADVANCED_FACE('',(#1825,#185),#1296,.T.);
#9852=ADVANCED_FACE('',(#1826),#9324,.T.);
#9853=ADVANCED_FACE('',(#1827),#1297,.F.);
#9854=ADVANCED_FACE('',(#1828,#186),#1298,.T.);
#9855=ADVANCED_FACE('',(#1829),#9325,.T.);
#9856=ADVANCED_FACE('',(#1830),#1299,.F.);
#9857=ADVANCED_FACE('',(#1831,#187),#1300,.T.);
#9858=ADVANCED_FACE('',(#1832),#9326,.T.);
#9859=ADVANCED_FACE('',(#1833),#1301,.F.);
#9860=ADVANCED_FACE('',(#1834,#188),#1302,.T.);
#9861=ADVANCED_FACE('',(#1835),#9327,.T.);
#9862=ADVANCED_FACE('',(#1836),#1303,.F.);
#9863=ADVANCED_FACE('',(#1837),#9328,.T.);
#9864=ADVANCED_FACE('',(#1838),#9329,.T.);
#9865=ADVANCED_FACE('',(#1839),#9330,.T.);
#9866=ADVANCED_FACE('',(#1840),#9331,.T.);
#9867=ADVANCED_FACE('',(#1841),#273,.F.);
#9868=ADVANCED_FACE('',(#1842),#9332,.T.);
#9869=ADVANCED_FACE('',(#1843),#274,.F.);
#9870=ADVANCED_FACE('',(#1844),#275,.F.);
#9871=ADVANCED_FACE('',(#1845),#276,.F.);
#9872=ADVANCED_FACE('',(#1846),#9333,.T.);
#9873=ADVANCED_FACE('',(#1847),#277,.F.);
#9874=ADVANCED_FACE('',(#1848),#278,.F.);
#9875=ADVANCED_FACE('',(#1849),#1304,.F.);
#9876=ADVANCED_FACE('',(#1850),#279,.F.);
#9877=ADVANCED_FACE('',(#1851),#280,.F.);
#9878=ADVANCED_FACE('',(#1852),#281,.F.);
#9879=ADVANCED_FACE('',(#1853,#189,#190),#1305,.T.);
#9880=ADVANCED_FACE('',(#1854),#1306,.F.);
#9881=ADVANCED_FACE('',(#1855),#282,.F.);
#9882=ADVANCED_FACE('',(#1856),#283,.F.);
#9883=ADVANCED_FACE('',(#1857,#191,#192,#193,#194,#195,#196),#1307,.F.);
#9884=ADVANCED_FACE('',(#1858),#284,.F.);
#9897=CLOSED_SHELL('',(#9849,#9850,#9851,#9852,#9853,#9854,#9855,#9856,
#9857,#9858,#9859,#9860,#9861,#9862,#9863,#9864,#9865,#9866,#9867,#9868,
#9869,#9870,#9871,#9872,#9873,#9874,#9875,#9876,#9877,#9878,#9879,#9880,
#9881,#9882,#9883,#9884));
#10595=AXIS2_PLACEMENT_3D('',#24166,#12413,#12414);
#10596=AXIS2_PLACEMENT_3D('',#24167,#12415,#12416);
#10597=AXIS2_PLACEMENT_3D('',#24169,#12417,#12418);
#10598=AXIS2_PLACEMENT_3D('',#24172,#12420,#12421);
#10599=AXIS2_PLACEMENT_3D('',#24173,#12422,#12423);
#10600=AXIS2_PLACEMENT_3D('',#24175,#12424,#12425);
#10601=AXIS2_PLACEMENT_3D('',#24178,#12427,#12428);
#10602=AXIS2_PLACEMENT_3D('',#24179,#12429,#12430);
#10603=AXIS2_PLACEMENT_3D('',#24181,#12431,#12432);
#10604=AXIS2_PLACEMENT_3D('',#24183,#12433,#12434);
#10605=AXIS2_PLACEMENT_3D('',#24184,#12435,#12436);
#10606=AXIS2_PLACEMENT_3D('',#24186,#12437,#12438);
#10607=AXIS2_PLACEMENT_3D('',#24188,#12440,#12441);
#10608=AXIS2_PLACEMENT_3D('',#24189,#12442,#12443);
#10609=AXIS2_PLACEMENT_3D('',#24191,#12444,#12445);
#10610=AXIS2_PLACEMENT_3D('',#24193,#12446,#12447);
#10611=AXIS2_PLACEMENT_3D('',#24194,#12448,#12449);
#10612=AXIS2_PLACEMENT_3D('',#24196,#12450,#12451);
#10613=AXIS2_PLACEMENT_3D('',#24198,#12453,#12454);
#10614=AXIS2_PLACEMENT_3D('',#24199,#12455,#12456);
#10615=AXIS2_PLACEMENT_3D('',#24201,#12457,#12458);
#10616=AXIS2_PLACEMENT_3D('',#24203,#12459,#12460);
#10617=AXIS2_PLACEMENT_3D('',#24204,#12461,#12462);
#10618=AXIS2_PLACEMENT_3D('',#24206,#12463,#12464);
#10619=AXIS2_PLACEMENT_3D('',#24208,#12466,#12467);
#10620=AXIS2_PLACEMENT_3D('',#24209,#12468,#12469);
#10621=AXIS2_PLACEMENT_3D('',#24211,#12470,#12471);
#10622=AXIS2_PLACEMENT_3D('',#24213,#12472,#12473);
#10623=AXIS2_PLACEMENT_3D('',#24214,#12474,#12475);
#10624=AXIS2_PLACEMENT_3D('',#24216,#12476,#12477);
#10625=AXIS2_PLACEMENT_3D('',#24218,#12479,#12480);
#10626=AXIS2_PLACEMENT_3D('',#24219,#12481,#12482);
#10627=AXIS2_PLACEMENT_3D('',#24222,#12484,#12485);
#10628=AXIS2_PLACEMENT_3D('',#24223,#12486,#12487);
#10629=AXIS2_PLACEMENT_3D('',#24226,#12489,#12490);
#10630=AXIS2_PLACEMENT_3D('',#24227,#12491,#12492);
#10631=AXIS2_PLACEMENT_3D('',#24230,#12494,#12495);
#10632=AXIS2_PLACEMENT_3D('',#24231,#12496,#12497);
#10633=AXIS2_PLACEMENT_3D('',#24234,#12499,#12500);
#10634=AXIS2_PLACEMENT_3D('',#24262,#12501,#12502);
#10635=AXIS2_PLACEMENT_3D('',#24270,#12503,#12504);
#10636=AXIS2_PLACEMENT_3D('',#24276,#12505,#12506);
#10637=AXIS2_PLACEMENT_3D('',#24279,#12507,#12508);
#10638=AXIS2_PLACEMENT_3D('',#24309,#12511,#12512);
#10639=AXIS2_PLACEMENT_3D('',#24347,#12513,#12514);
#10640=AXIS2_PLACEMENT_3D('',#24385,#12515,#12516);
#10641=AXIS2_PLACEMENT_3D('',#24396,#12517,#12518);
#10642=AXIS2_PLACEMENT_3D('',#24399,#12519,#12520);
#10643=AXIS2_PLACEMENT_3D('',#24429,#12523,#12524);
#10644=AXIS2_PLACEMENT_3D('',#24475,#12525,#12526);
#10645=AXIS2_PLACEMENT_3D('',#24618,#12528,#12529);
#10646=AXIS2_PLACEMENT_3D('',#24619,#12530,#12531);
#10647=AXIS2_PLACEMENT_3D('',#24732,#12533,#12534);
#12413=DIRECTION('axis',(0.,0.,1.));
#12414=DIRECTION('refdir',(1.,0.,0.));
#12415=DIRECTION('center_axis',(0.,0.,-1.));
#12416=DIRECTION('ref_axis',(1.,0.,0.));
#12417=DIRECTION('center_axis',(1.16928610669829E-31,-5.97538301968883E-32,
-1.));
#12418=DIRECTION('ref_axis',(1.,0.,0.));
#12419=DIRECTION('',(0.,0.,-1.));
#12420=DIRECTION('center_axis',(-6.45616000593692E-32,-1.81182428107391E-19,
1.));
#12421=DIRECTION('ref_axis',(1.,0.,0.));
#12422=DIRECTION('center_axis',(0.,0.,-1.));
#12423=DIRECTION('ref_axis',(1.,0.,0.));
#12424=DIRECTION('center_axis',(1.16928610669829E-31,-5.97538301968883E-32,
-1.));
#12425=DIRECTION('ref_axis',(1.,0.,0.));
#12426=DIRECTION('',(0.,0.,-1.));
#12427=DIRECTION('center_axis',(-6.45616000593692E-32,-1.81182428107391E-19,
1.));
#12428=DIRECTION('ref_axis',(1.,0.,0.));
#12429=DIRECTION('center_axis',(0.,0.,1.));
#12430=DIRECTION('ref_axis',(1.,0.,0.));
#12431=DIRECTION('center_axis',(0.,0.,1.));
#12432=DIRECTION('ref_axis',(1.,0.,0.));
#12433=DIRECTION('center_axis',(0.,0.,-1.));
#12434=DIRECTION('ref_axis',(1.,0.,0.));
#12435=DIRECTION('center_axis',(0.,0.,-1.));
#12436=DIRECTION('ref_axis',(1.,0.,0.));
#12437=DIRECTION('center_axis',(0.,0.,-1.));
#12438=DIRECTION('ref_axis',(1.,0.,0.));
#12439=DIRECTION('',(0.,0.,1.));
#12440=DIRECTION('center_axis',(0.,0.,1.));
#12441=DIRECTION('ref_axis',(1.,0.,0.));
#12442=DIRECTION('center_axis',(0.,0.,1.));
#12443=DIRECTION('ref_axis',(1.,0.,0.));
#12444=DIRECTION('center_axis',(0.,0.,1.));
#12445=DIRECTION('ref_axis',(1.,0.,0.));
#12446=DIRECTION('center_axis',(0.,0.,-1.));
#12447=DIRECTION('ref_axis',(1.,0.,0.));
#12448=DIRECTION('center_axis',(0.,0.,-1.));
#12449=DIRECTION('ref_axis',(1.,0.,0.));
#12450=DIRECTION('center_axis',(0.,0.,-1.));
#12451=DIRECTION('ref_axis',(1.,0.,0.));
#12452=DIRECTION('',(0.,0.,1.));
#12453=DIRECTION('center_axis',(0.,0.,1.));
#12454=DIRECTION('ref_axis',(1.,0.,0.));
#12455=DIRECTION('center_axis',(0.,0.,1.));
#12456=DIRECTION('ref_axis',(1.,0.,0.));
#12457=DIRECTION('center_axis',(0.,0.,1.));
#12458=DIRECTION('ref_axis',(1.,0.,0.));
#12459=DIRECTION('center_axis',(0.,0.,-1.));
#12460=DIRECTION('ref_axis',(1.,0.,0.));
#12461=DIRECTION('center_axis',(0.,0.,-1.));
#12462=DIRECTION('ref_axis',(1.,0.,0.));
#12463=DIRECTION('center_axis',(0.,0.,-1.));
#12464=DIRECTION('ref_axis',(1.,0.,0.));
#12465=DIRECTION('',(0.,0.,1.));
#12466=DIRECTION('center_axis',(0.,0.,1.));
#12467=DIRECTION('ref_axis',(1.,0.,0.));
#12468=DIRECTION('center_axis',(0.,0.,1.));
#12469=DIRECTION('ref_axis',(1.,0.,0.));
#12470=DIRECTION('center_axis',(0.,0.,1.));
#12471=DIRECTION('ref_axis',(1.,0.,0.));
#12472=DIRECTION('center_axis',(0.,0.,-1.));
#12473=DIRECTION('ref_axis',(1.,0.,0.));
#12474=DIRECTION('center_axis',(0.,0.,-1.));
#12475=DIRECTION('ref_axis',(1.,0.,0.));
#12476=DIRECTION('center_axis',(0.,0.,-1.));
#12477=DIRECTION('ref_axis',(1.,0.,0.));
#12478=DIRECTION('',(0.,0.,1.));
#12479=DIRECTION('center_axis',(0.,0.,1.));
#12480=DIRECTION('ref_axis',(1.,0.,0.));
#12481=DIRECTION('center_axis',(0.,0.,-1.));
#12482=DIRECTION('ref_axis',(1.,0.,0.));
#12483=DIRECTION('',(0.,0.,1.));
#12484=DIRECTION('center_axis',(-6.45616000593692E-32,-1.81182428107391E-19,
1.));
#12485=DIRECTION('ref_axis',(1.,0.,0.));
#12486=DIRECTION('center_axis',(0.,0.,-1.));
#12487=DIRECTION('ref_axis',(1.,0.,0.));
#12488=DIRECTION('',(0.,0.,1.));
#12489=DIRECTION('center_axis',(-6.45616000593692E-32,-1.81182428107391E-19,
1.));
#12490=DIRECTION('ref_axis',(1.,0.,0.));
#12491=DIRECTION('center_axis',(0.,0.,-1.));
#12492=DIRECTION('ref_axis',(1.,0.,0.));
#12493=DIRECTION('',(0.,0.,1.));
#12494=DIRECTION('center_axis',(-6.45616000593692E-32,-1.81182428107391E-19,
1.));
#12495=DIRECTION('ref_axis',(1.,0.,0.));
#12496=DIRECTION('center_axis',(0.,0.,-1.));
#12497=DIRECTION('ref_axis',(1.,0.,0.));
#12498=DIRECTION('',(0.,0.,1.));
#12499=DIRECTION('center_axis',(-6.45616000593692E-32,-1.81182428107391E-19,
1.));
#12500=DIRECTION('ref_axis',(1.,0.,0.));
#12501=DIRECTION('center_axis',(0.,1.,0.));
#12502=DIRECTION('ref_axis',(0.,0.,1.));
#12503=DIRECTION('center_axis',(0.998287351281347,-0.0585009766728139,0.));
#12504=DIRECTION('ref_axis',(0.0584117362954384,0.996764512774636,0.0552139034672828));
#12505=DIRECTION('center_axis',(-3.13156554427463E-33,-1.,5.97538301968883E-32));
#12506=DIRECTION('ref_axis',(0.688354575693766,0.,0.725374371012276));
#12507=DIRECTION('center_axis',(1.38968329343724E-15,1.,0.));
#12508=DIRECTION('ref_axis',(0.,0.,1.));
#12509=DIRECTION('',(3.13156554427463E-33,1.,-5.97538301968883E-32));
#12510=DIRECTION('',(-3.13156554427463E-33,-1.,5.97538301968883E-32));
#12511=DIRECTION('center_axis',(0.998287351281345,0.0585009766728351,0.));
#12512=DIRECTION('ref_axis',(0.,0.,1.));
#12513=DIRECTION('center_axis',(0.996325437245183,-0.0856482521607663,0.));
#12514=DIRECTION('ref_axis',(0.,0.,1.));
#12515=DIRECTION('center_axis',(-1.38968329343725E-15,-1.,-6.75000545323542E-30));
#12516=DIRECTION('ref_axis',(-4.85722573273506E-15,0.,1.));
#12517=DIRECTION('center_axis',(-3.13156554427485E-33,1.,-5.97538301968883E-32));
#12518=DIRECTION('ref_axis',(-0.688354575693752,0.,0.72537437101229));
#12519=DIRECTION('center_axis',(1.38968329343726E-15,-1.,0.));
#12520=DIRECTION('ref_axis',(0.,0.,1.));
#12521=DIRECTION('',(3.13156554427485E-33,-1.,5.97538301968883E-32));
#12522=DIRECTION('',(-3.13156554427485E-33,1.,-5.97538301968883E-32));
#12523=DIRECTION('center_axis',(-0.996325437245184,-0.0856482521607654,
-4.83937755196581E-15));
#12524=DIRECTION('ref_axis',(-4.85722573273506E-15,0.,1.));
#12525=DIRECTION('center_axis',(0.998629534754574,0.,-0.0523359562429439));
#12526=DIRECTION('ref_axis',(-0.0523359562429439,0.,-0.998629534754574));
#12527=DIRECTION('',(0.,1.,0.));
#12528=DIRECTION('center_axis',(-1.16928610669829E-31,5.97538301968883E-32,
1.));
#12529=DIRECTION('ref_axis',(1.,0.,1.16928610669829E-31));
#12530=DIRECTION('center_axis',(-0.998629534754574,0.,-0.0523359562429402));
#12531=DIRECTION('ref_axis',(-0.0523359562429402,0.,0.998629534754574));
#12532=DIRECTION('',(0.,-1.,0.));
#12533=DIRECTION('center_axis',(-6.45616000593692E-32,-1.81182428107391E-19,
1.));
#12534=DIRECTION('ref_axis',(1.,0.,6.45616000593692E-32));
#24166=CARTESIAN_POINT('',(0.,0.,0.));
#24167=CARTESIAN_POINT('Origin',(2.,0.,1.));
#24168=CARTESIAN_POINT('',(1.65,4.28626379701574E-17,1.1));
#24169=CARTESIAN_POINT('Origin',(2.,0.,1.1));
#24170=CARTESIAN_POINT('',(1.65,4.28626379701574E-17,0.9));
#24171=CARTESIAN_POINT('',(1.65,4.28626379701574E-17,1.));
#24172=CARTESIAN_POINT('Origin',(2.,0.,0.9));
#24173=CARTESIAN_POINT('Origin',(8.8,0.,1.));
#24174=CARTESIAN_POINT('',(8.45,4.28626379701574E-17,1.1));
#24175=CARTESIAN_POINT('Origin',(8.8,0.,1.1));
#24176=CARTESIAN_POINT('',(8.45,4.28626379701574E-17,0.9));
#24177=CARTESIAN_POINT('',(8.45,4.28626379701574E-17,1.));
#24178=CARTESIAN_POINT('Origin',(8.8,0.,0.9));
#24179=CARTESIAN_POINT('Origin',(8.1,1.,0.7));
#24180=CARTESIAN_POINT('',(7.85,1.,0.7));
#24181=CARTESIAN_POINT('Origin',(8.1,1.,0.7));
#24182=CARTESIAN_POINT('',(7.95,1.,0.7));
#24183=CARTESIAN_POINT('Origin',(8.1,1.,0.7));
#24184=CARTESIAN_POINT('Origin',(8.1,1.,0.7));
#24185=CARTESIAN_POINT('',(7.85,1.,0.6));
#24186=CARTESIAN_POINT('Origin',(8.1,1.,0.6));
#24187=CARTESIAN_POINT('',(7.85,1.,0.7));
#24188=CARTESIAN_POINT('Origin',(8.1,1.,0.6));
#24189=CARTESIAN_POINT('Origin',(2.7,-1.,0.7));
#24190=CARTESIAN_POINT('',(2.45,-1.,0.7));
#24191=CARTESIAN_POINT('Origin',(2.7,-1.,0.7));
#24192=CARTESIAN_POINT('',(2.55,-1.,0.7));
#24193=CARTESIAN_POINT('Origin',(2.7,-1.,0.7));
#24194=CARTESIAN_POINT('Origin',(2.7,-1.,0.7));
#24195=CARTESIAN_POINT('',(2.45,-1.,0.6));
#24196=CARTESIAN_POINT('Origin',(2.7,-1.,0.6));
#24197=CARTESIAN_POINT('',(2.45,-1.,0.7));
#24198=CARTESIAN_POINT('Origin',(2.7,-1.,0.6));
#24199=CARTESIAN_POINT('Origin',(2.7,1.,0.7));
#24200=CARTESIAN_POINT('',(2.45,1.,0.7));
#24201=CARTESIAN_POINT('Origin',(2.7,1.,0.7));
#24202=CARTESIAN_POINT('',(2.55,1.,0.7));
#24203=CARTESIAN_POINT('Origin',(2.7,1.,0.7));
#24204=CARTESIAN_POINT('Origin',(2.7,1.,0.7));
#24205=CARTESIAN_POINT('',(2.45,1.,0.6));
#24206=CARTESIAN_POINT('Origin',(2.7,1.,0.6));
#24207=CARTESIAN_POINT('',(2.45,1.,0.7));
#24208=CARTESIAN_POINT('Origin',(2.7,1.,0.6));
#24209=CARTESIAN_POINT('Origin',(8.1,-1.,0.7));
#24210=CARTESIAN_POINT('',(7.85,-1.,0.7));
#24211=CARTESIAN_POINT('Origin',(8.1,-1.,0.7));
#24212=CARTESIAN_POINT('',(7.95,-1.,0.7));
#24213=CARTESIAN_POINT('Origin',(8.1,-1.,0.7));
#24214=CARTESIAN_POINT('Origin',(8.1,-1.,0.7));
#24215=CARTESIAN_POINT('',(7.85,-1.,0.6));
#24216=CARTESIAN_POINT('Origin',(8.1,-1.,0.6));
#24217=CARTESIAN_POINT('',(7.85,-1.,0.7));
#24218=CARTESIAN_POINT('Origin',(8.1,-1.,0.6));
#24219=CARTESIAN_POINT('Origin',(8.1,1.,0.9));
#24220=CARTESIAN_POINT('',(7.95,1.,0.9));
#24221=CARTESIAN_POINT('',(7.95,1.,0.9));
#24222=CARTESIAN_POINT('Origin',(8.1,1.,0.9));
#24223=CARTESIAN_POINT('Origin',(2.7,-1.,0.9));
#24224=CARTESIAN_POINT('',(2.55,-1.,0.9));
#24225=CARTESIAN_POINT('',(2.55,-1.,0.9));
#24226=CARTESIAN_POINT('Origin',(2.7,-1.,0.9));
#24227=CARTESIAN_POINT('Origin',(2.7,1.,0.9));
#24228=CARTESIAN_POINT('',(2.55,1.,0.9));
#24229=CARTESIAN_POINT('',(2.55,1.,0.9));
#24230=CARTESIAN_POINT('Origin',(2.7,1.,0.9));
#24231=CARTESIAN_POINT('Origin',(8.1,-1.,0.9));
#24232=CARTESIAN_POINT('',(7.95,-1.,0.9));
#24233=CARTESIAN_POINT('',(7.95,-1.,0.9));
#24234=CARTESIAN_POINT('Origin',(8.1,-1.,0.9));
#24235=CARTESIAN_POINT('Ctrl Pts',(10.3006295894369,0.974894988741159,1.1));
#24236=CARTESIAN_POINT('Ctrl Pts',(10.315705472156,0.974011521809381,1.1));
#24237=CARTESIAN_POINT('Ctrl Pts',(10.3502474882039,0.960160784532573,1.1));
#24238=CARTESIAN_POINT('Ctrl Pts',(10.3664342774515,0.92524659453289,1.1));
#24239=CARTESIAN_POINT('Ctrl Pts',(10.3664342774515,0.905110932257975,1.1));
#24240=CARTESIAN_POINT('Ctrl Pts',(10.3019806204244,0.997949597787003,1.1));
#24241=CARTESIAN_POINT('Ctrl Pts',(10.3220349090938,0.996609784625678,1.09999398337427));
#24242=CARTESIAN_POINT('Ctrl Pts',(10.3677183242066,0.978025516808524,1.09998506712737));
#24243=CARTESIAN_POINT('Ctrl Pts',(10.3893396302527,0.931918448901421,1.09999143472557));
#24244=CARTESIAN_POINT('Ctrl Pts',(10.3895723566779,0.905110932257975,1.1));
#24245=CARTESIAN_POINT('Ctrl Pts',(10.3043223099121,1.03790925537118,1.08136572286424));
#24246=CARTESIAN_POINT('Ctrl Pts',(10.3329503749445,1.0358015962555,1.08164234815929));
#24247=CARTESIAN_POINT('Ctrl Pts',(10.3979372989902,1.00899285190124,1.08203919297574));
#24248=CARTESIAN_POINT('Ctrl Pts',(10.4290660105163,0.943405843911333,1.08168333012239));
#24249=CARTESIAN_POINT('Ctrl Pts',(10.4296737498558,0.905110932257975,1.08129070628762));
#24250=CARTESIAN_POINT('Ctrl Pts',(10.3052465815697,1.05368144854439,1.04171131144128));
#24251=CARTESIAN_POINT('Ctrl Pts',(10.3373036016374,1.05157771141627,1.04242733672965));
#24252=CARTESIAN_POINT('Ctrl Pts',(10.4104769365187,1.02185126978705,1.04346621563788));
#24253=CARTESIAN_POINT('Ctrl Pts',(10.445100550936,0.94795146444073,1.04253150017828));
#24254=CARTESIAN_POINT('Ctrl Pts',(10.4454164251054,0.905110932257975,1.0415166534692));
#24255=CARTESIAN_POINT('Ctrl Pts',(10.3053025283406,1.05463614976313,1.02441711227736));
#24256=CARTESIAN_POINT('Ctrl Pts',(10.3375636805833,1.05269876817044,1.02526261130878));
#24257=CARTESIAN_POINT('Ctrl Pts',(10.411517621087,1.0229540574362,1.02649649899074));
#24258=CARTESIAN_POINT('Ctrl Pts',(10.4462618831994,0.948196125723061,1.02538435201347));
#24259=CARTESIAN_POINT('Ctrl Pts',(10.4463246402318,0.905110932257975,1.02418687649944));
#24260=CARTESIAN_POINT('',(10.3664342774515,0.905110932257975,1.1));
#24261=CARTESIAN_POINT('',(10.4463246402318,0.905110932257975,1.02418687649943));
#24262=CARTESIAN_POINT('Origin',(10.3664342774515,0.905110932257975,1.02));
#24263=CARTESIAN_POINT('',(10.3053025283406,1.05463614976313,1.02441711227738));
#24264=CARTESIAN_POINT('Ctrl Pts',(10.4463246402318,0.905110932257975,1.02418687649944));
#24265=CARTESIAN_POINT('Ctrl Pts',(10.4462618831994,0.948196125723061,1.02538435201347));
#24266=CARTESIAN_POINT('Ctrl Pts',(10.411517621087,1.0229540574362,1.02649649899074));
#24267=CARTESIAN_POINT('Ctrl Pts',(10.3375636805833,1.05269876817044,1.02526261130878));
#24268=CARTESIAN_POINT('Ctrl Pts',(10.3053025283406,1.05463614976313,1.02441711227736));
#24269=CARTESIAN_POINT('',(10.3006295894369,0.974894988741159,1.1));
#24270=CARTESIAN_POINT('Origin',(10.3006295894369,0.974894988741159,1.02));
#24271=CARTESIAN_POINT('Ctrl Pts',(10.3006295894369,0.974894988741159,1.1));
#24272=CARTESIAN_POINT('Ctrl Pts',(10.315705472156,0.974011521809381,1.1));
#24273=CARTESIAN_POINT('Ctrl Pts',(10.3502474882039,0.960160784532573,1.1));
#24274=CARTESIAN_POINT('Ctrl Pts',(10.3664342774515,0.92524659453289,1.1));
#24275=CARTESIAN_POINT('Ctrl Pts',(10.3664342774515,0.905110932257975,1.1));
#24276=CARTESIAN_POINT('Origin',(10.3664342774515,0.526416499322631,1.02));
#24277=CARTESIAN_POINT('',(10.3664342774515,-0.905110932257974,1.1));
#24278=CARTESIAN_POINT('',(10.4463246402318,-0.905110932257974,1.02418687649944));
#24279=CARTESIAN_POINT('Origin',(10.3664342774515,-0.905110932257974,1.02));
#24280=CARTESIAN_POINT('',(10.4463246402318,0.526416499322631,1.02418687649944));
#24281=CARTESIAN_POINT('',(10.3664342774515,0.526416499322631,1.1));
#24282=CARTESIAN_POINT('Ctrl Pts',(10.3664342774515,-0.905110932257974,
1.1));
#24283=CARTESIAN_POINT('Ctrl Pts',(10.3664342774515,-0.920212678972614,
1.1));
#24284=CARTESIAN_POINT('Ctrl Pts',(10.3546350195413,-0.955507038097987,
1.1));
#24285=CARTESIAN_POINT('Ctrl Pts',(10.3207307664069,-0.973717032831462,
1.1));
#24286=CARTESIAN_POINT('Ctrl Pts',(10.3006295894369,-0.974894988741159,
1.1));
#24287=CARTESIAN_POINT('Ctrl Pts',(10.3895723566779,-0.905110932257974,
1.1));
#24288=CARTESIAN_POINT('Ctrl Pts',(10.3893978118589,-0.925216569751813,
1.09999357604418));
#24289=CARTESIAN_POINT('Ctrl Pts',(10.3734893817427,-0.971910228734234,
1.09998467394719));
#24290=CARTESIAN_POINT('Ctrl Pts',(10.3287196719985,-0.996163180237569,
1.09999197783236));
#24291=CARTESIAN_POINT('Ctrl Pts',(10.3019806204244,-0.997949597787003,
1.1));
#24292=CARTESIAN_POINT('Ctrl Pts',(10.4296737498558,-0.905110932257974,
1.0812907062876));
#24293=CARTESIAN_POINT('Ctrl Pts',(10.4292179453509,-0.933832116014069,
1.08158517416384));
#24294=CARTESIAN_POINT('Ctrl Pts',(10.4061705706524,-1.00027633256302,1.08203447943735));
#24295=CARTESIAN_POINT('Ctrl Pts',(10.3424930633099,-1.03509904321534,1.08173455659116));
#24296=CARTESIAN_POINT('Ctrl Pts',(10.3043223099121,-1.03790925537115,1.08136572286421));
#24297=CARTESIAN_POINT('Ctrl Pts',(10.4454164251054,-0.905110932257974,
1.0415166534692));
#24298=CARTESIAN_POINT('Ctrl Pts',(10.4451795194782,-0.937241331413026,
1.04227778850144));
#24299=CARTESIAN_POINT('Ctrl Pts',(10.4197512278104,-1.01202259423409,1.0434534732467));
#24300=CARTESIAN_POINT('Ctrl Pts',(10.3479892750172,-1.05087646570533,1.0426660118263));
#24301=CARTESIAN_POINT('Ctrl Pts',(10.3052465815697,-1.05368144854438,1.04171131144128));
#24302=CARTESIAN_POINT('Ctrl Pts',(10.4463246402318,-0.905110932257974,
1.02418687649944));
#24303=CARTESIAN_POINT('Ctrl Pts',(10.4462775724575,-0.937424827374877,
1.02508498313546));
#24304=CARTESIAN_POINT('Ctrl Pts',(10.4209202812412,-1.01298254961426,1.02648109501254));
#24305=CARTESIAN_POINT('Ctrl Pts',(10.3483173980216,-1.05205297430477,1.02554444431988));
#24306=CARTESIAN_POINT('Ctrl Pts',(10.3053025283406,-1.05463614976313,1.02441711227736));
#24307=CARTESIAN_POINT('',(10.3006295894369,-0.974894988741159,1.1));
#24308=CARTESIAN_POINT('',(10.3053025283406,-1.05463614976313,1.02441711227736));
#24309=CARTESIAN_POINT('Origin',(10.3006295894369,-0.974894988741159,1.02));
#24310=CARTESIAN_POINT('Ctrl Pts',(10.3053025283406,-1.05463614976313,1.02441711227736));
#24311=CARTESIAN_POINT('Ctrl Pts',(10.3483173980216,-1.05205297430477,1.02554444431988));
#24312=CARTESIAN_POINT('Ctrl Pts',(10.4209202812412,-1.01298254961426,1.02648109501254));
#24313=CARTESIAN_POINT('Ctrl Pts',(10.4462775724575,-0.937424827374877,
1.02508498313546));
#24314=CARTESIAN_POINT('Ctrl Pts',(10.4463246402318,-0.905110932257974,
1.02418687649944));
#24315=CARTESIAN_POINT('Ctrl Pts',(10.3664342774515,-0.905110932257974,
1.1));
#24316=CARTESIAN_POINT('Ctrl Pts',(10.3664342774515,-0.920212678972614,
1.1));
#24317=CARTESIAN_POINT('Ctrl Pts',(10.3546350195413,-0.955507038097987,
1.1));
#24318=CARTESIAN_POINT('Ctrl Pts',(10.3207307664069,-0.973717032831462,
1.1));
#24319=CARTESIAN_POINT('Ctrl Pts',(10.3006295894369,-0.974894988741159,
1.1));
#24320=CARTESIAN_POINT('Ctrl Pts',(10.3006295894369,-0.974894988741159,
1.1));
#24321=CARTESIAN_POINT('Ctrl Pts',(8.90133038997308,-1.05689579714676,1.1));
#24322=CARTESIAN_POINT('Ctrl Pts',(5.63386529032775,-1.20659234980357,1.1));
#24323=CARTESIAN_POINT('Ctrl Pts',(2.35953432096223,-1.1387902266302,1.1));
#24324=CARTESIAN_POINT('Ctrl Pts',(0.497468741075922,-0.978719373910683,
1.1));
#24325=CARTESIAN_POINT('Ctrl Pts',(10.3019806204244,-0.997949597787003,
1.1));
#24326=CARTESIAN_POINT('Ctrl Pts',(8.90248440956766,-1.07998148241326,1.10000071389857));
#24327=CARTESIAN_POINT('Ctrl Pts',(5.63428345559727,-1.22975661509925,1.09999860206726));
#24328=CARTESIAN_POINT('Ctrl Pts',(2.35854977485598,-1.16192218645588,1.10000206853834));
#24329=CARTESIAN_POINT('Ctrl Pts',(0.495492436783665,-1.00170924455528,
1.1));
#24330=CARTESIAN_POINT('Ctrl Pts',(10.3043223112023,-1.03790927738781,1.08136574244164));
#24331=CARTESIAN_POINT('Ctrl Pts',(8.90448672538924,-1.11999254202045,1.08133291965814));
#24332=CARTESIAN_POINT('Ctrl Pts',(5.63501252140964,-1.26990499402305,1.08126385742935));
#24333=CARTESIAN_POINT('Ctrl Pts',(2.35683262246169,-1.20200947624765,1.08130376582018));
#24334=CARTESIAN_POINT('Ctrl Pts',(0.492066872450609,-1.0415580073244,1.08139899772624));
#24335=CARTESIAN_POINT('Ctrl Pts',(10.3052465815697,-1.05368144854439,1.04171131144128));
#24336=CARTESIAN_POINT('Ctrl Pts',(8.90527383415966,-1.13574844311122,1.04162635195479));
#24337=CARTESIAN_POINT('Ctrl Pts',(5.63529344743191,-1.28563363803111,1.04144655753461));
#24338=CARTESIAN_POINT('Ctrl Pts',(2.35616768559357,-1.21776439538312,1.04155103737704));
#24339=CARTESIAN_POINT('Ctrl Pts',(0.490711556403977,-1.05732407164794,
1.04179769276967));
#24340=CARTESIAN_POINT('Ctrl Pts',(10.3053025283406,-1.05463614976313,1.02441711227736));
#24341=CARTESIAN_POINT('Ctrl Pts',(8.90532084970199,-1.13668250951809,1.02431679017323));
#24342=CARTESIAN_POINT('Ctrl Pts',(5.63530902077156,-1.28652517622799,1.02410366945797));
#24343=CARTESIAN_POINT('Ctrl Pts',(2.35612886002319,-1.2186808487933,1.02422798328229));
#24344=CARTESIAN_POINT('Ctrl Pts',(0.490627822843887,-1.05829812393464,
1.02451933428366));
#24345=CARTESIAN_POINT('',(0.497468741075922,-0.978719373910683,1.1));
#24346=CARTESIAN_POINT('',(0.490627822843887,-1.05829812393464,1.02451933428366));
#24347=CARTESIAN_POINT('Origin',(0.497468741075922,-0.978719373910683,1.02));
#24348=CARTESIAN_POINT('Ctrl Pts',(0.490627822843887,-1.05829812393464,
1.02451933428366));
#24349=CARTESIAN_POINT('Ctrl Pts',(2.35612886002319,-1.2186808487933,1.02422798328229));
#24350=CARTESIAN_POINT('Ctrl Pts',(5.63530902077156,-1.28652517622799,1.02410366945797));
#24351=CARTESIAN_POINT('Ctrl Pts',(8.90532084970199,-1.13668250951809,1.02431679017323));
#24352=CARTESIAN_POINT('Ctrl Pts',(10.3053025283406,-1.05463614976313,1.02441711227736));
#24353=CARTESIAN_POINT('Ctrl Pts',(10.3006295894369,-0.974894988741159,
1.1));
#24354=CARTESIAN_POINT('Ctrl Pts',(8.90133038997308,-1.05689579714676,1.1));
#24355=CARTESIAN_POINT('Ctrl Pts',(5.63386529032775,-1.20659234980357,1.1));
#24356=CARTESIAN_POINT('Ctrl Pts',(2.35953432096223,-1.1387902266302,1.1));
#24357=CARTESIAN_POINT('Ctrl Pts',(0.497468741075922,-0.978719373910683,
1.1));
#24358=CARTESIAN_POINT('Ctrl Pts',(0.497468741075921,-0.978719373910683,
1.1));
#24359=CARTESIAN_POINT('Ctrl Pts',(0.482693827936028,-0.977449261315989,
1.1));
#24360=CARTESIAN_POINT('Ctrl Pts',(0.449140492346353,-0.963153189418853,
1.1));
#24361=CARTESIAN_POINT('Ctrl Pts',(0.433565722548535,-0.928845297374623,
1.1));
#24362=CARTESIAN_POINT('Ctrl Pts',(0.433565722548535,-0.909072757750428,
1.1));
#24363=CARTESIAN_POINT('Ctrl Pts',(0.495492436783665,-1.00170924455528,
1.1));
#24364=CARTESIAN_POINT('Ctrl Pts',(0.475845599502289,-0.99986336234735,
1.09999428725696));
#24365=CARTESIAN_POINT('Ctrl Pts',(0.431470670910625,-0.980707626108276,
1.09998595101222));
#24366=CARTESIAN_POINT('Ctrl Pts',(0.410656014536328,-0.935396857641307,
1.09999159501496));
#24367=CARTESIAN_POINT('Ctrl Pts',(0.410427643322096,-0.909072757750428,
1.1));
#24368=CARTESIAN_POINT('Ctrl Pts',(0.49206544526959,-1.04157460937658,1.08141381101793));
#24369=CARTESIAN_POINT('Ctrl Pts',(0.464027324938814,-1.03875422423143,
1.08167681576789));
#24370=CARTESIAN_POINT('Ctrl Pts',(0.40089609645214,-1.01114975683443,1.0820463630617));
#24371=CARTESIAN_POINT('Ctrl Pts',(0.370905720538455,-0.946677133941945,
1.08169093175476));
#24372=CARTESIAN_POINT('Ctrl Pts',(0.370309354350992,-0.909072757750428,
1.08130565542949));
#24373=CARTESIAN_POINT('Ctrl Pts',(0.490711556403977,-1.05732407164794,
1.04179769276967));
#24374=CARTESIAN_POINT('Ctrl Pts',(0.459302109313527,-1.05440855600651,
1.04247888820671));
#24375=CARTESIAN_POINT('Ctrl Pts',(0.388222412631637,-1.02376232464153,
1.04344633806995));
#24376=CARTESIAN_POINT('Ctrl Pts',(0.354893537837358,-0.951140796546497,
1.04251250847383));
#24377=CARTESIAN_POINT('Ctrl Pts',(0.354583574894625,-0.909072757750428,
1.0415166534692));
#24378=CARTESIAN_POINT('Ctrl Pts',(0.490627822843887,-1.05829812393464,
1.02451933428366));
#24379=CARTESIAN_POINT('Ctrl Pts',(0.45900946369528,-1.05553438344805,1.02532396689517));
#24380=CARTESIAN_POINT('Ctrl Pts',(0.387169680965019,-1.0248398620393,1.02647307310763));
#24381=CARTESIAN_POINT('Ctrl Pts',(0.353736942373964,-0.951381046565093,
1.02536194261819));
#24382=CARTESIAN_POINT('Ctrl Pts',(0.35367535976817,-0.909072757750428,
1.02418687649944));
#24383=CARTESIAN_POINT('',(0.433565722548535,-0.909072757750428,1.1));
#24384=CARTESIAN_POINT('',(0.35367535976817,-0.909072757750428,1.02418687649944));
#24385=CARTESIAN_POINT('Origin',(0.433565722548536,-0.909072757750428,1.02));
#24386=CARTESIAN_POINT('Ctrl Pts',(0.35367535976817,-0.909072757750428,
1.02418687649944));
#24387=CARTESIAN_POINT('Ctrl Pts',(0.353736942373964,-0.951381046565093,
1.02536194261819));
#24388=CARTESIAN_POINT('Ctrl Pts',(0.387169680965019,-1.0248398620393,1.02647307310763));
#24389=CARTESIAN_POINT('Ctrl Pts',(0.45900946369528,-1.05553438344805,1.02532396689517));
#24390=CARTESIAN_POINT('Ctrl Pts',(0.490627822843887,-1.05829812393464,
1.02451933428366));
#24391=CARTESIAN_POINT('Ctrl Pts',(0.497468741075921,-0.978719373910683,
1.1));
#24392=CARTESIAN_POINT('Ctrl Pts',(0.482693827936028,-0.977449261315989,
1.1));
#24393=CARTESIAN_POINT('Ctrl Pts',(0.449140492346353,-0.963153189418853,
1.1));
#24394=CARTESIAN_POINT('Ctrl Pts',(0.433565722548535,-0.928845297374623,
1.1));
#24395=CARTESIAN_POINT('Ctrl Pts',(0.433565722548535,-0.909072757750428,
1.1));
#24396=CARTESIAN_POINT('Origin',(0.433565722548535,-0.526416499322631,1.02));
#24397=CARTESIAN_POINT('',(0.433565722548535,0.909072757750428,1.1));
#24398=CARTESIAN_POINT('',(0.35367535976817,0.909072757750428,1.02418687649944));
#24399=CARTESIAN_POINT('Origin',(0.433565722548535,0.909072757750428,1.02));
#24400=CARTESIAN_POINT('',(0.35367535976817,-0.526416499322631,1.02418687649944));
#24401=CARTESIAN_POINT('',(0.433565722548535,-0.526416499322631,1.1));
#24402=CARTESIAN_POINT('Ctrl Pts',(0.433565722548535,0.909072757750428,
1.1));
#24403=CARTESIAN_POINT('Ctrl Pts',(0.433565722548535,0.923902162481473,
1.1));
#24404=CARTESIAN_POINT('Ctrl Pts',(0.444925688709976,0.95855828847753,1.1));
#24405=CARTESIAN_POINT('Ctrl Pts',(0.477768856872262,0.977025890449618,
1.1));
#24406=CARTESIAN_POINT('Ctrl Pts',(0.497468741075921,0.978719373910683,
1.1));
#24407=CARTESIAN_POINT('Ctrl Pts',(0.410427643322096,0.909072757750428,
1.1));
#24408=CARTESIAN_POINT('Ctrl Pts',(0.410598921732919,0.928815832685761,
1.09999369626122));
#24409=CARTESIAN_POINT('Ctrl Pts',(0.425924740546693,0.974670094016788,
1.09998538828789));
#24410=CARTESIAN_POINT('Ctrl Pts',(0.469296653719045,0.9992480682759,1.09999238300928));
#24411=CARTESIAN_POINT('Ctrl Pts',(0.495492436783665,1.00170924455528,1.1));
#24412=CARTESIAN_POINT('Ctrl Pts',(0.370309354350991,0.909072757750428,
1.08130565542949));
#24413=CARTESIAN_POINT('Ctrl Pts',(0.370756628991978,0.937276039918598,
1.0815946126737));
#24414=CARTESIAN_POINT('Ctrl Pts',(0.392976709797646,1.00253976529927,1.08203966084696));
#24415=CARTESIAN_POINT('Ctrl Pts',(0.454681284796039,1.03781409584644,1.08176448401818));
#24416=CARTESIAN_POINT('Ctrl Pts',(0.49206544526959,1.04157460937658,1.08141381101793));
#24417=CARTESIAN_POINT('Ctrl Pts',(0.354583574894625,0.909072757750428,
1.0415166534692));
#24418=CARTESIAN_POINT('Ctrl Pts',(0.354816047101877,0.940623786874923,
1.04226354472332));
#24419=CARTESIAN_POINT('Ctrl Pts',(0.379310481833935,1.01405872099116,1.04342813304911));
#24420=CARTESIAN_POINT('Ctrl Pts',(0.448832293580284,1.05343671745598,1.04270595335318));
#24421=CARTESIAN_POINT('Ctrl Pts',(0.490711556403977,1.05732407164794,1.04179769276967));
#24422=CARTESIAN_POINT('Ctrl Pts',(0.35367535976817,0.909072757750428,1.02418687649944));
#24423=CARTESIAN_POINT('Ctrl Pts',(0.353721546722556,0.940803974389028,
1.02506817608927));
#24424=CARTESIAN_POINT('Ctrl Pts',(0.378136805744942,1.01499479618886,1.02645106984513));
#24425=CARTESIAN_POINT('Ctrl Pts',(0.448470010609076,1.05461313661598,1.0255921777666));
#24426=CARTESIAN_POINT('Ctrl Pts',(0.490627822843887,1.05829812393464,1.02451933428366));
#24427=CARTESIAN_POINT('',(0.497468741075921,0.978719373910683,1.1));
#24428=CARTESIAN_POINT('',(0.490627822843887,1.05829812393464,1.02451933428366));
#24429=CARTESIAN_POINT('Origin',(0.497468741075921,0.978719373910683,1.02));
#24430=CARTESIAN_POINT('Ctrl Pts',(0.490627822843887,1.05829812393464,1.02451933428366));
#24431=CARTESIAN_POINT('Ctrl Pts',(0.448470010609076,1.05461313661598,1.0255921777666));
#24432=CARTESIAN_POINT('Ctrl Pts',(0.378136805744942,1.01499479618886,1.02645106984513));
#24433=CARTESIAN_POINT('Ctrl Pts',(0.353721546722556,0.940803974389028,
1.02506817608927));
#24434=CARTESIAN_POINT('Ctrl Pts',(0.35367535976817,0.909072757750428,1.02418687649944));
#24435=CARTESIAN_POINT('Ctrl Pts',(0.433565722548535,0.909072757750428,
1.1));
#24436=CARTESIAN_POINT('Ctrl Pts',(0.433565722548535,0.923902162481473,
1.1));
#24437=CARTESIAN_POINT('Ctrl Pts',(0.444925688709976,0.95855828847753,1.1));
#24438=CARTESIAN_POINT('Ctrl Pts',(0.477768856872262,0.977025890449618,
1.1));
#24439=CARTESIAN_POINT('Ctrl Pts',(0.497468741075921,0.978719373910683,
1.1));
#24440=CARTESIAN_POINT('Ctrl Pts',(0.497468741075922,0.978719373910683,
1.1));
#24441=CARTESIAN_POINT('Ctrl Pts',(1.89401780684616,1.09877250320817,1.1));
#24442=CARTESIAN_POINT('Ctrl Pts',(5.1654052076905,1.21987569230965,1.1));
#24443=CARTESIAN_POINT('Ctrl Pts',(8.43489748265729,1.08422939062092,1.1));
#24444=CARTESIAN_POINT('Ctrl Pts',(10.3006295894369,0.974894988741159,1.1));
#24445=CARTESIAN_POINT('Ctrl Pts',(0.495492436783665,1.00170924455528,1.1));
#24446=CARTESIAN_POINT('Ctrl Pts',(1.89278532112995,1.12186894072949,1.10000155140362));
#24447=CARTESIAN_POINT('Ctrl Pts',(5.16566149651331,1.24305592512388,1.09999870932828));
#24448=CARTESIAN_POINT('Ctrl Pts',(8.43598583180997,1.1073254346241,1.10000095186468));
#24449=CARTESIAN_POINT('Ctrl Pts',(10.3019806204244,0.997949597787003,1.1));
#24450=CARTESIAN_POINT('Ctrl Pts',(0.492066872450609,1.0415580073244,1.08139899772624));
#24451=CARTESIAN_POINT('Ctrl Pts',(1.89064106564166,1.16189659875033,1.08132757380279));
#24452=CARTESIAN_POINT('Ctrl Pts',(5.16610832342906,1.28323142649893,1.0812556832418));
#24453=CARTESIAN_POINT('Ctrl Pts',(8.43787502268472,1.14735362089424,1.08132197873404));
#24454=CARTESIAN_POINT('Ctrl Pts',(10.3043223112023,1.03790927738781,1.08136574244164));
#24455=CARTESIAN_POINT('Ctrl Pts',(0.490711556403977,1.05732407164794,1.04179769276967));
#24456=CARTESIAN_POINT('Ctrl Pts',(1.88980353393473,1.17765430418353,1.04161270124098));
#24457=CARTESIAN_POINT('Ctrl Pts',(5.16628155123749,1.29896165650174,1.04142536433641));
#24458=CARTESIAN_POINT('Ctrl Pts',(8.43861641093843,1.16310409863161,1.04159803213562));
#24459=CARTESIAN_POINT('Ctrl Pts',(10.3052465815697,1.05368144854439,1.04171131144128));
#24460=CARTESIAN_POINT('Ctrl Pts',(0.490627822843887,1.05829812393464,1.02451933428366));
#24461=CARTESIAN_POINT('Ctrl Pts',(1.88975348136405,1.17858515731652,1.02430082105127));
#24462=CARTESIAN_POINT('Ctrl Pts',(5.16629169073646,1.29984841142479,1.02407861909595));
#24463=CARTESIAN_POINT('Ctrl Pts',(8.43866044940558,1.1640312867702,1.02428334948326));
#24464=CARTESIAN_POINT('Ctrl Pts',(10.3053025283406,1.05463614976313,1.02441711227736));
#24465=CARTESIAN_POINT('Ctrl Pts',(10.3053025283406,1.05463614976313,1.02441711227736));
#24466=CARTESIAN_POINT('Ctrl Pts',(8.43866044940558,1.1640312867702,1.02428334948326));
#24467=CARTESIAN_POINT('Ctrl Pts',(5.16629169073646,1.29984841142479,1.02407861909595));
#24468=CARTESIAN_POINT('Ctrl Pts',(1.88975348136405,1.17858515731652,1.02430082105127));
#24469=CARTESIAN_POINT('Ctrl Pts',(0.490627822843887,1.05829812393464,1.02451933428366));
#24470=CARTESIAN_POINT('Ctrl Pts',(0.497468741075922,0.978719373910683,
1.1));
#24471=CARTESIAN_POINT('Ctrl Pts',(1.89401780684616,1.09877250320817,1.1));
#24472=CARTESIAN_POINT('Ctrl Pts',(5.1654052076905,1.21987569230965,1.1));
#24473=CARTESIAN_POINT('Ctrl Pts',(8.43489748265729,1.08422939062092,1.1));
#24474=CARTESIAN_POINT('Ctrl Pts',(10.3006295894369,0.974894988741159,1.1));
#24475=CARTESIAN_POINT('Origin',(0.347167001354737,-1.05283299864526,0.9));
#24476=CARTESIAN_POINT('',(0.347167001354737,0.915565952400859,0.9));
#24477=CARTESIAN_POINT('Ctrl Pts',(0.347167001354737,0.915565952400859,
0.9));
#24478=CARTESIAN_POINT('Ctrl Pts',(0.349336454142569,0.913401548092598,
0.941395625182189));
#24479=CARTESIAN_POINT('Ctrl Pts',(0.351505906947026,0.911237149868421,
0.982791250681617));
#24480=CARTESIAN_POINT('Ctrl Pts',(0.35367535976817,0.909072757750428,1.02418687649944));
#24481=CARTESIAN_POINT('',(0.347167001354737,-0.915565952400859,0.9));
#24482=CARTESIAN_POINT('',(0.347167001354737,-1.05283299864526,0.9));
#24483=CARTESIAN_POINT('Ctrl Pts',(0.35367535976817,-0.909072757750428,
1.02418687649944));
#24484=CARTESIAN_POINT('Ctrl Pts',(0.351505906947026,-0.911237149868421,
0.982791250681617));
#24485=CARTESIAN_POINT('Ctrl Pts',(0.349336454142569,-0.913401548092598,
0.941395625182188));
#24486=CARTESIAN_POINT('Ctrl Pts',(0.347167001354737,-0.915565952400859,
0.9));
#24487=CARTESIAN_POINT('Ctrl Pts',(0.346993933238254,0.915738617787778,
0.896697663613103));
#24488=CARTESIAN_POINT('Ctrl Pts',(0.349221075397351,0.913516658022686,
0.939194067573829));
#24489=CARTESIAN_POINT('Ctrl Pts',(0.351448217573968,0.911294704668933,
0.981690471868858));
#24490=CARTESIAN_POINT('Ctrl Pts',(0.35367535976817,0.909072757750428,1.02418687649944));
#24491=CARTESIAN_POINT('Ctrl Pts',(0.3471095194732,0.958036394339727,0.898903180361322));
#24492=CARTESIAN_POINT('Ctrl Pts',(0.349336694827029,0.955813381999015,
0.941399523267081));
#24493=CARTESIAN_POINT('Ctrl Pts',(0.351563761373338,0.953590428181058,
0.983895874971514));
#24494=CARTESIAN_POINT('Ctrl Pts',(0.353790936839104,0.951367426011707,
1.0263922183879));
#24495=CARTESIAN_POINT('Ctrl Pts',(0.38058410360499,1.03143776743275,0.900986703480571));
#24496=CARTESIAN_POINT('Ctrl Pts',(0.382809509257377,1.02921304595835,0.943483042387942));
#24497=CARTESIAN_POINT('Ctrl Pts',(0.38503494445329,1.0269883029847,0.985979378580875));
#24498=CARTESIAN_POINT('Ctrl Pts',(0.38726034587086,1.02476358729949,1.02847571797107));
#24499=CARTESIAN_POINT('Ctrl Pts',(0.452370958194108,1.06215086202928,0.898830373501354));
#24500=CARTESIAN_POINT('Ctrl Pts',(0.454593549384999,1.0599273359084,0.941326919294252));
#24501=CARTESIAN_POINT('Ctrl Pts',(0.456816159498039,1.05770384366995,0.983823465869045));
#24502=CARTESIAN_POINT('Ctrl Pts',(0.459038739297573,1.0554803259981,1.02632001264655));
#24503=CARTESIAN_POINT('Ctrl Pts',(0.48397786901498,1.06495020962439,0.897320291708494));
#24504=CARTESIAN_POINT('Ctrl Pts',(0.486199596570706,1.06272777115298,0.939816939358577));
#24505=CARTESIAN_POINT('Ctrl Pts',(0.488421317286976,1.06050533819043,0.982313587627294));
#24506=CARTESIAN_POINT('Ctrl Pts',(0.49064303113777,1.05828291075608,1.02481023651688));
#24507=CARTESIAN_POINT('',(0.484117964332956,1.06481006947648,0.9));
#24508=CARTESIAN_POINT('Ctrl Pts',(0.490627822843887,1.05829812393464,1.02451933428366));
#24509=CARTESIAN_POINT('Ctrl Pts',(0.488457876548035,1.06046876718106,0.983012888930867));
#24510=CARTESIAN_POINT('Ctrl Pts',(0.486287923702977,1.06263941570101,0.941506444170341));
#24511=CARTESIAN_POINT('Ctrl Pts',(0.484117964332956,1.06481006947648,0.9));
#24512=CARTESIAN_POINT('Ctrl Pts',(0.484117964332956,1.06481006947648,0.9));
#24513=CARTESIAN_POINT('Ctrl Pts',(0.473400395954556,1.06388989254567,0.899999999998067));
#24514=CARTESIAN_POINT('Ctrl Pts',(0.462835544435656,1.06178983909504,0.899998456484708));
#24515=CARTESIAN_POINT('Ctrl Pts',(0.452598733053303,1.05860868771556,0.899998088469989));
#24516=CARTESIAN_POINT('Ctrl Pts',(0.444242646677269,1.05601198306707,0.899997788067582));
#24517=CARTESIAN_POINT('Ctrl Pts',(0.436104524303727,1.05269365102958,0.899998236040192));
#24518=CARTESIAN_POINT('Ctrl Pts',(0.428287607266336,1.04868302953039,0.899999222960128));
#24519=CARTESIAN_POINT('Ctrl Pts',(0.418720381516706,1.0437743780639,0.900000430864189));
#24520=CARTESIAN_POINT('Ctrl Pts',(0.409734998843702,1.03788190267505,0.900002558923036));
#24521=CARTESIAN_POINT('Ctrl Pts',(0.401509364000825,1.03108161209803,0.900001877425249));
#24522=CARTESIAN_POINT('Ctrl Pts',(0.400282968007853,1.0300677269361,0.900001775817754));
#24523=CARTESIAN_POINT('Ctrl Pts',(0.399073506836177,1.02903357975146,0.900001605039306));
#24524=CARTESIAN_POINT('Ctrl Pts',(0.397881626738084,1.02797933950107,0.900001345423406));
#24525=CARTESIAN_POINT('Ctrl Pts',(0.39256805719391,1.02327938780652,0.900000188019117));
#24526=CARTESIAN_POINT('Ctrl Pts',(0.387603264903844,1.01818054769329,0.899997323013939));
#24527=CARTESIAN_POINT('Ctrl Pts',(0.383010638913681,1.01272978836618,0.899994456107983));
#24528=CARTESIAN_POINT('Ctrl Pts',(0.37606924632558,1.00449139480359,0.899990123005355));
#24529=CARTESIAN_POINT('Ctrl Pts',(0.370046554889952,0.995534526609835,
0.899986018340436));
#24530=CARTESIAN_POINT('Ctrl Pts',(0.3650033874046,0.986038739193365,0.899984773108821));
#24531=CARTESIAN_POINT('Ctrl Pts',(0.361794276996282,0.979996300523246,
0.899983980732651));
#24532=CARTESIAN_POINT('Ctrl Pts',(0.358982518390177,0.973734765189587,
0.899984261914926));
#24533=CARTESIAN_POINT('Ctrl Pts',(0.356593362150852,0.967295151176304,
0.899985518247832));
#24534=CARTESIAN_POINT('Ctrl Pts',(0.352862932284158,0.957240334312622,
0.899987479886722));
#24535=CARTESIAN_POINT('Ctrl Pts',(0.350196128254646,0.946848238515865,
0.899991935314924));
#24536=CARTESIAN_POINT('Ctrl Pts',(0.348668140386249,0.936282377262574,
0.899995621109591));
#24537=CARTESIAN_POINT('Ctrl Pts',(0.347678076093379,0.929436195976283,
0.89999800933123));
#24538=CARTESIAN_POINT('Ctrl Pts',(0.347167001781036,0.922516504287414,
0.899999999966543));
#24539=CARTESIAN_POINT('Ctrl Pts',(0.347167001354737,0.915565952400859,
0.9));
#24540=CARTESIAN_POINT('Ctrl Pts',(0.484117964332956,1.06481006947648,0.9));
#24541=CARTESIAN_POINT('Ctrl Pts',(0.486234267105876,1.06263480888061,0.94150644476122));
#24542=CARTESIAN_POINT('Ctrl Pts',(0.488350569878795,1.06045954828474,0.98301288952244));
#24543=CARTESIAN_POINT('Ctrl Pts',(0.490466872651714,1.05828428768887,1.02451933428366));
#24544=CARTESIAN_POINT('Ctrl Pts',(3.76001591476243,1.34606837492147,0.9));
#24545=CARTESIAN_POINT('Ctrl Pts',(3.76072193310094,1.3438931143256,0.94150644476122));
#24546=CARTESIAN_POINT('Ctrl Pts',(3.76142795143945,1.34171785372973,0.98301288952244));
#24547=CARTESIAN_POINT('Ctrl Pts',(3.76213396977796,1.33954259313386,1.02451933428366));
#24548=CARTESIAN_POINT('Ctrl Pts',(7.03591386519191,1.25287427294368,0.9));
#24549=CARTESIAN_POINT('Ctrl Pts',(7.03520959909601,1.25069901234781,0.94150644476122));
#24550=CARTESIAN_POINT('Ctrl Pts',(7.03450533300011,1.24852375175194,0.98301288952244));
#24551=CARTESIAN_POINT('Ctrl Pts',(7.03380106690421,1.24634849115607,1.02451933428366));
#24552=CARTESIAN_POINT('Ctrl Pts',(10.3118118156214,1.06114656258054,0.9));
#24553=CARTESIAN_POINT('Ctrl Pts',(10.3096972650911,1.05897130198467,0.94150644476122));
#24554=CARTESIAN_POINT('Ctrl Pts',(10.3075827145608,1.0567960413888,0.98301288952244));
#24555=CARTESIAN_POINT('Ctrl Pts',(10.3054681640305,1.05462078079293,1.02451933428366));
#24556=CARTESIAN_POINT('',(10.3118118156214,1.06114656258054,0.9));
#24557=CARTESIAN_POINT('Ctrl Pts',(10.3118118156214,1.06114656258054,0.9));
#24558=CARTESIAN_POINT('Ctrl Pts',(10.3096420485163,1.05897642099582,0.941472370325488));
#24559=CARTESIAN_POINT('Ctrl Pts',(10.3074722860834,1.05680628338526,0.982944741084089));
#24560=CARTESIAN_POINT('Ctrl Pts',(10.3053025283406,1.05463614976313,1.02441711227738));
#24561=CARTESIAN_POINT('Ctrl Pts',(0.484117964332956,1.06481006947648,0.9));
#24562=CARTESIAN_POINT('Ctrl Pts',(3.76001591476244,1.34606837492147,0.9));
#24563=CARTESIAN_POINT('Ctrl Pts',(7.03591386519191,1.25287427294368,0.9));
#24564=CARTESIAN_POINT('Ctrl Pts',(10.3118118156214,1.06114656258054,0.9));
#24565=CARTESIAN_POINT('Ctrl Pts',(10.3119584735067,1.0612932457764,0.897196819041737));
#24566=CARTESIAN_POINT('Ctrl Pts',(10.3097363069231,1.05907069570186,0.939670735378922));
#24567=CARTESIAN_POINT('Ctrl Pts',(10.3075141452397,1.0568481497954,0.982144652170355));
#24568=CARTESIAN_POINT('Ctrl Pts',(10.3052919884757,1.05462560807237,1.02461856941773));
#24569=CARTESIAN_POINT('Ctrl Pts',(10.3549577591382,1.05865952187103,0.899312513938921));
#24570=CARTESIAN_POINT('Ctrl Pts',(10.3527348026837,1.05643589667682,0.941786332790264));
#24571=CARTESIAN_POINT('Ctrl Pts',(10.3505118643323,1.05421236578444,0.984260157591605));
#24572=CARTESIAN_POINT('Ctrl Pts',(10.348288915563,1.05198874626302,1.02673397710222));
#24573=CARTESIAN_POINT('Ctrl Pts',(10.427476572305,1.0195555601276,0.90106705940868));
#24574=CARTESIAN_POINT('Ctrl Pts',(10.4252515051274,1.01733143721131,0.943540744474557));
#24575=CARTESIAN_POINT('Ctrl Pts',(10.423026434404,1.01510729429004,0.986014428272043));
#24576=CARTESIAN_POINT('Ctrl Pts',(10.4208013694594,1.01288317591826,1.02848811366363));
#24577=CARTESIAN_POINT('Ctrl Pts',(10.452914163627,0.944082648463888,0.89845127988914));
#24578=CARTESIAN_POINT('Ctrl Pts',(10.4506882024692,0.941859792143813,0.940924989850352));
#24579=CARTESIAN_POINT('Ctrl Pts',(10.4484622663099,0.939636927142988,0.983398700650476));
#24580=CARTESIAN_POINT('Ctrl Pts',(10.4462363051112,0.937414078664829,1.02587241101113));
#24581=CARTESIAN_POINT('Ctrl Pts',(10.453002503567,0.911777874403687,0.896765653419433));
#24582=CARTESIAN_POINT('Ctrl Pts',(10.4507765491346,0.909555555737009,0.939239394205133));
#24583=CARTESIAN_POINT('Ctrl Pts',(10.4485505946895,0.90733324168256,0.981713135231494));
#24584=CARTESIAN_POINT('Ctrl Pts',(10.4463246402318,0.905110932257975,1.02418687649944));
#24585=CARTESIAN_POINT('',(10.4528329986453,0.911608646352005,0.9));
#24586=CARTESIAN_POINT('Ctrl Pts',(10.4463246402318,0.905110932257975,1.02418687649944));
#24587=CARTESIAN_POINT('Ctrl Pts',(10.4484940930483,0.90727683256362,0.982791250770435));
#24588=CARTESIAN_POINT('Ctrl Pts',(10.4506635458528,0.909442737267073,0.941395625270907));
#24589=CARTESIAN_POINT('Ctrl Pts',(10.4528329986453,0.911608646352005,0.9));
#24590=CARTESIAN_POINT('Ctrl Pts',(10.4528329986453,0.911608646352005,0.9));
#24591=CARTESIAN_POINT('Ctrl Pts',(10.4528329984504,0.922365992175136,0.899999999995018));
#24592=CARTESIAN_POINT('Ctrl Pts',(10.4516419184466,0.933071221555305,0.899998396191737));
#24593=CARTESIAN_POINT('Ctrl Pts',(10.4493455883239,0.943542152407774,0.899997878793429));
#24594=CARTESIAN_POINT('Ctrl Pts',(10.4474685729764,0.952101068966945,0.899997455873155));
#24595=CARTESIAN_POINT('Ctrl Pts',(10.4448518647823,0.96050416098414,0.899997731911133));
#24596=CARTESIAN_POINT('Ctrl Pts',(10.4415172538375,0.968646108261598,0.899998556768105));
#24597=CARTESIAN_POINT('Ctrl Pts',(10.4374420364703,0.978596355981088,0.899999564823172));
#24598=CARTESIAN_POINT('Ctrl Pts',(10.4323389624922,0.988051909949456,0.900001510869465));
#24599=CARTESIAN_POINT('Ctrl Pts',(10.4262707314398,0.996829854811629,0.900000879982417));
#24600=CARTESIAN_POINT('Ctrl Pts',(10.4250393574459,0.998611087749148,0.900000751961929));
#24601=CARTESIAN_POINT('Ctrl Pts',(10.4237680854757,1.0003643483506,0.900000505994341));
#24602=CARTESIAN_POINT('Ctrl Pts',(10.4224572101159,1.00208797543426,0.90000009374416));
#24603=CARTESIAN_POINT('Ctrl Pts',(10.4185057422955,1.00728363107359,0.899998851068177));
#24604=CARTESIAN_POINT('Ctrl Pts',(10.4141947510749,1.0122104380758,0.899996136506224));
#24605=CARTESIAN_POINT('Ctrl Pts',(10.4095592300387,1.01684760353016,0.899993329936423));
#24606=CARTESIAN_POINT('Ctrl Pts',(10.4019420261375,1.02446750958049,0.899988718110854));
#24607=CARTESIAN_POINT('Ctrl Pts',(10.3935294957569,1.03122853977634,0.899984126639313));
#24608=CARTESIAN_POINT('Ctrl Pts',(10.3844977038391,1.03705893037027,0.899982514537369));
#24609=CARTESIAN_POINT('Ctrl Pts',(10.3781912117148,1.04113002863034,0.899981388879436));
#24610=CARTESIAN_POINT('Ctrl Pts',(10.3715817027072,1.04474676663118,0.899981626398985));
#24611=CARTESIAN_POINT('Ctrl Pts',(10.364720849853,1.04787222446317,0.899983147799038));
#24612=CARTESIAN_POINT('Ctrl Pts',(10.3549611185069,1.05231826483487,0.899985312027903));
#24613=CARTESIAN_POINT('Ctrl Pts',(10.34479058664,1.05572789097839,0.899990169054599));
#24614=CARTESIAN_POINT('Ctrl Pts',(10.3343672593286,1.0580160164031,0.899994394012168));
#24615=CARTESIAN_POINT('Ctrl Pts',(10.3269595157814,1.05964216185967,0.899997396642827));
#24616=CARTESIAN_POINT('Ctrl Pts',(10.3194233385871,1.06070108442786,0.899999999979614));
#24617=CARTESIAN_POINT('Ctrl Pts',(10.3118118156214,1.06114656258054,0.9));
#24618=CARTESIAN_POINT('Origin',(5.4,6.06940689584926E-17,1.1));
#24619=CARTESIAN_POINT('Origin',(10.4528329986453,1.05283299864526,0.9));
#24620=CARTESIAN_POINT('',(10.4528329986453,-0.911608646352005,0.9));
#24621=CARTESIAN_POINT('Ctrl Pts',(10.4528329986453,-0.911608646352005,
0.9));
#24622=CARTESIAN_POINT('Ctrl Pts',(10.4506635458528,-0.909442737267072,
0.941395625270908));
#24623=CARTESIAN_POINT('Ctrl Pts',(10.4484940930483,-0.90727683256362,0.982791250770435));
#24624=CARTESIAN_POINT('Ctrl Pts',(10.4463246402318,-0.905110932257974,
1.02418687649944));
#24625=CARTESIAN_POINT('',(10.4528329986453,1.05283299864526,0.9));
#24626=CARTESIAN_POINT('Ctrl Pts',(0.483981659460312,-1.06494641796617,
0.897392794396587));
#24627=CARTESIAN_POINT('Ctrl Pts',(0.486202123526484,-1.0627252433871,0.939865274484676));
#24628=CARTESIAN_POINT('Ctrl Pts',(0.488422580760962,-1.06050407431064,
0.982337755190696));
#24629=CARTESIAN_POINT('Ctrl Pts',(0.49064303113777,-1.05828291075608,1.02481023651688));
#24630=CARTESIAN_POINT('Ctrl Pts',(0.441839113682364,-1.06121395205434,
0.899406236555586));
#24631=CARTESIAN_POINT('Ctrl Pts',(0.444060746976072,-1.05899130022525,
0.941878578466899));
#24632=CARTESIAN_POINT('Ctrl Pts',(0.446282352620465,-1.05676877539366,
0.984350928552248));
#24633=CARTESIAN_POINT('Ctrl Pts',(0.448503975350841,-1.05454613107877,
1.02682327135645));
#24634=CARTESIAN_POINT('Ctrl Pts',(0.371552730979752,-1.02159229167772,
0.901018138383736));
#24635=CARTESIAN_POINT('Ctrl Pts',(0.373777362914204,-1.01936901231721,
0.943490294374253));
#24636=CARTESIAN_POINT('Ctrl Pts',(0.376002007910301,-1.01714569791452,
0.985962447794501));
#24637=CARTESIAN_POINT('Ctrl Pts',(0.378226636819208,-1.01492242480963,
1.02843460423251));
#24638=CARTESIAN_POINT('Ctrl Pts',(0.347084422593646,-0.947458158036175,
0.898424303372123));
#24639=CARTESIAN_POINT('Ctrl Pts',(0.349310306978605,-0.945236691937326,
0.940896495998715));
#24640=CARTESIAN_POINT('Ctrl Pts',(0.351536158132471,-0.943015214174121,
0.983368689735046));
#24641=CARTESIAN_POINT('Ctrl Pts',(0.353762042571371,-0.940793758946387,
1.02584088291578));
#24642=CARTESIAN_POINT('Ctrl Pts',(0.346997732921341,-0.915734826946278,
0.896770165885443));
#24643=CARTESIAN_POINT('Ctrl Pts',(0.349223608519428,-0.913514130802309,
0.939242402422435));
#24644=CARTESIAN_POINT('Ctrl Pts',(0.351449484135017,-0.911293441062403,
0.981714639293352));
#24645=CARTESIAN_POINT('Ctrl Pts',(0.35367535976817,-0.909072757750428,
1.02418687649944));
#24646=CARTESIAN_POINT('',(0.484117964332957,-1.06481006947648,0.9));
#24647=CARTESIAN_POINT('Ctrl Pts',(0.347167001354737,-0.915565952400859,
0.9));
#24648=CARTESIAN_POINT('Ctrl Pts',(0.347167001618251,-0.926324952789844,
0.899999999993398));
#24649=CARTESIAN_POINT('Ctrl Pts',(0.348355267190738,-0.937032860435638,
0.899998616841383));
#24650=CARTESIAN_POINT('Ctrl Pts',(0.350648507770679,-0.947506517879914,
0.899998360166273));
#24651=CARTESIAN_POINT('Ctrl Pts',(0.352522341068277,-0.956064664041459,
0.899998150434084));
#24652=CARTESIAN_POINT('Ctrl Pts',(0.355135157141203,-0.964467130383873,
0.899998666502847));
#24653=CARTESIAN_POINT('Ctrl Pts',(0.358466575399326,-0.972608174091076,
0.89999965996049));
#24654=CARTESIAN_POINT('Ctrl Pts',(0.362538734686669,-0.982559379305286,
0.900000874313493));
#24655=CARTESIAN_POINT('Ctrl Pts',(0.367640276064737,-0.992015301694373,
0.90000291775694));
#24656=CARTESIAN_POINT('Ctrl Pts',(0.373711018494534,-1.00079214745216,
0.900002098461893));
#24657=CARTESIAN_POINT('Ctrl Pts',(0.3746124109217,-1.00209534593109,0.900001976811805));
#24658=CARTESIAN_POINT('Ctrl Pts',(0.375535256028145,-1.00338353399439,
0.900001785555943));
#24659=CARTESIAN_POINT('Ctrl Pts',(0.376479443106529,-1.00465606108108,
0.900001505529245));
#24660=CARTESIAN_POINT('Ctrl Pts',(0.380715143239362,-1.01036472123276,
0.900000249306668));
#24661=CARTESIAN_POINT('Ctrl Pts',(0.38537983051291,-1.01575881671377,0.899997265714102));
#24662=CARTESIAN_POINT('Ctrl Pts',(0.390428509023093,-1.02081078987204,
0.899994288896867));
#24663=CARTESIAN_POINT('Ctrl Pts',(0.398043974952909,-1.02843122547465,
0.899989798642598));
#24664=CARTESIAN_POINT('Ctrl Pts',(0.406453848296673,-1.0351976329321,0.899985566096));
#24665=CARTESIAN_POINT('Ctrl Pts',(0.415484607049401,-1.04103374418621,
0.899984276342262));
#24666=CARTESIAN_POINT('Ctrl Pts',(0.421222938370041,-1.04474213026064,
0.899983456806));
#24667=CARTESIAN_POINT('Ctrl Pts',(0.427212893823217,-1.04807424787086,
0.899983742291921));
#24668=CARTESIAN_POINT('Ctrl Pts',(0.433415948881005,-1.05100146303553,
0.899985033489932));
#24669=CARTESIAN_POINT('Ctrl Pts',(0.443112479013355,-1.05557724541753,
0.899987051872858));
#24670=CARTESIAN_POINT('Ctrl Pts',(0.453235937005982,-1.05912207412747,
0.899991654125809));
#24671=CARTESIAN_POINT('Ctrl Pts',(0.463629957379397,-1.06154692150368,
0.899995467994069));
#24672=CARTESIAN_POINT('Ctrl Pts',(0.470358492676306,-1.06311663856929,
0.899997936889288));
#24673=CARTESIAN_POINT('Ctrl Pts',(0.477201035001208,-1.06421620326297,
0.899999999975707));
#24674=CARTESIAN_POINT('Ctrl Pts',(0.484117964332956,-1.06481006947648,
0.9));
#24675=CARTESIAN_POINT('Ctrl Pts',(0.484117964332957,-1.06481006947648,
0.9));
#24676=CARTESIAN_POINT('Ctrl Pts',(0.486287923702977,-1.06263941570101,
0.941506444170342));
#24677=CARTESIAN_POINT('Ctrl Pts',(0.488457876548035,-1.06046876718106,
0.983012888930867));
#24678=CARTESIAN_POINT('Ctrl Pts',(0.490627822843887,-1.05829812393464,
1.02451933428366));
#24679=CARTESIAN_POINT('Ctrl Pts',(10.453005262311,-0.911780628641664,0.896713013448579));
#24680=CARTESIAN_POINT('Ctrl Pts',(10.4507783882972,-0.909557391891849,
0.939204300891032));
#24681=CARTESIAN_POINT('Ctrl Pts',(10.4485515142709,-0.907334159758067,
0.981695588574342));
#24682=CARTESIAN_POINT('Ctrl Pts',(10.4463246402318,-0.905110932257974,
1.02418687649944));
#24683=CARTESIAN_POINT('Ctrl Pts',(10.4528874757217,-0.954853661617317,
0.898960515458773));
#24684=CARTESIAN_POINT('Ctrl Pts',(10.4506605772126,-0.952629688741643,
0.941451759962203));
#24685=CARTESIAN_POINT('Ctrl Pts',(10.4484337586651,-0.950405759674027,
0.983943010977281));
#24686=CARTESIAN_POINT('Ctrl Pts',(10.4462068600709,-0.94818179413378,1.02643425584837));
#24687=CARTESIAN_POINT('Ctrl Pts',(10.4180804799687,-1.02952167699519,0.901043151378083));
#24688=CARTESIAN_POINT('Ctrl Pts',(10.4158548456208,-1.02729651565793,0.943534394542847));
#24689=CARTESIAN_POINT('Ctrl Pts',(10.413629193759,-1.02507134540722,0.986025636297673));
#24690=CARTESIAN_POINT('Ctrl Pts',(10.4114035625395,-1.02284618829514,1.02851687981561));
#24691=CARTESIAN_POINT('Ctrl Pts',(10.3442106925096,-1.05932070834318,0.898730950115076));
#24692=CARTESIAN_POINT('Ctrl Pts',(10.3419870251366,-1.05709644901815,0.941222341385074));
#24693=CARTESIAN_POINT('Ctrl Pts',(10.3397633429135,-1.0548722146549,0.983713733185165));
#24694=CARTESIAN_POINT('Ctrl Pts',(10.3375396837912,-1.05264796171536,1.0262051251811));
#24695=CARTESIAN_POINT('Ctrl Pts',(10.3119612275562,-1.06129600030118,0.897144178853313));
#24696=CARTESIAN_POINT('Ctrl Pts',(10.309738142952,-1.05907253204827,0.939635641919598));
#24697=CARTESIAN_POINT('Ctrl Pts',(10.3075150632522,-1.05684906796687,0.982127105440503));
#24698=CARTESIAN_POINT('Ctrl Pts',(10.3052919884757,-1.05462560807237,1.02461856941773));
#24699=CARTESIAN_POINT('',(10.3118118156214,-1.06114656258054,0.9));
#24700=CARTESIAN_POINT('Ctrl Pts',(10.3053025283406,-1.05463614976313,1.02441711227736));
#24701=CARTESIAN_POINT('Ctrl Pts',(10.3074722860834,-1.05680628338526,0.982944741084074));
#24702=CARTESIAN_POINT('Ctrl Pts',(10.3096420485163,-1.05897642099582,0.941472370325482));
#24703=CARTESIAN_POINT('Ctrl Pts',(10.3118118156214,-1.06114656258054,0.900000000000001));
#24704=CARTESIAN_POINT('Ctrl Pts',(10.3118118156214,-1.06114656258054,0.900000000000001));
#24705=CARTESIAN_POINT('Ctrl Pts',(10.322549369014,-1.06051812817027,0.899999999998837));
#24706=CARTESIAN_POINT('Ctrl Pts',(10.3331651969327,-1.05870347076406,0.899998279675625));
#24707=CARTESIAN_POINT('Ctrl Pts',(10.3434824690201,-1.05579899810317,0.899997678781422));
#24708=CARTESIAN_POINT('Ctrl Pts',(10.3519099591122,-1.05342652848477,0.899997187951103));
#24709=CARTESIAN_POINT('Ctrl Pts',(10.3601388923794,-1.05032564389788,0.899997411230107));
#24710=CARTESIAN_POINT('Ctrl Pts',(10.368065652211,-1.04652424300033,0.899998227267474));
#24711=CARTESIAN_POINT('Ctrl Pts',(10.3777613500057,-1.04187452040475,0.89999922541197));
#24712=CARTESIAN_POINT('Ctrl Pts',(10.3869029298231,-1.0362271920453,0.900001226887481));
#24713=CARTESIAN_POINT('Ctrl Pts',(10.3953114913929,-1.02965576012812,0.900000692598515));
#24714=CARTESIAN_POINT('Ctrl Pts',(10.3970212347867,-1.0283195669856,0.900000583959597));
#24715=CARTESIAN_POINT('Ctrl Pts',(10.3987005924826,-1.02694501523934,0.900000358370781));
#24716=CARTESIAN_POINT('Ctrl Pts',(10.4003479139729,-1.02553250004787,0.899999966744969));
#24717=CARTESIAN_POINT('Ctrl Pts',(10.4052955867552,-1.02129005981461,0.899998790510468));
#24718=CARTESIAN_POINT('Ctrl Pts',(10.4099546972526,-1.01670546321193,0.899996154952331));
#24719=CARTESIAN_POINT('Ctrl Pts',(10.4143066574475,-1.01181472964029,0.899993423989004));
#24720=CARTESIAN_POINT('Ctrl Pts',(10.4214686344271,-1.00376609875091,0.899988929670213));
#24721=CARTESIAN_POINT('Ctrl Pts',(10.4277268376922,-0.994973664259554,
0.899984438878373));
#24722=CARTESIAN_POINT('Ctrl Pts',(10.4330201329469,-0.985617486073369,
0.899982870029797));
#24723=CARTESIAN_POINT('Ctrl Pts',(10.4367196060238,-0.979078472540647,
0.89998177356478));
#24724=CARTESIAN_POINT('Ctrl Pts',(10.4399470827666,-0.972263038755175,
0.89998201356482));
#24725=CARTESIAN_POINT('Ctrl Pts',(10.4426687152005,-0.965225084739993,
0.899983510148066));
#24726=CARTESIAN_POINT('Ctrl Pts',(10.4465375225522,-0.955220615401818,
0.899985637544916));
#24727=CARTESIAN_POINT('Ctrl Pts',(10.4493477346146,-0.944866529467853,
0.899990392295554));
#24728=CARTESIAN_POINT('Ctrl Pts',(10.4510237312406,-0.934325606572895,
0.899994522211612));
#24729=CARTESIAN_POINT('Ctrl Pts',(10.452215546318,-0.926829869027476,0.899997459029114));
#24730=CARTESIAN_POINT('Ctrl Pts',(10.452832998309,-0.919238945488459,0.899999999973399));
#24731=CARTESIAN_POINT('Ctrl Pts',(10.4528329986453,-0.911608646352004,
0.9));
#24732=CARTESIAN_POINT('Origin',(5.4,0.,0.9));
#24733=CARTESIAN_POINT('Ctrl Pts',(10.3118118156214,-1.06114656258054,0.9));
#24734=CARTESIAN_POINT('Ctrl Pts',(7.03591386519191,-1.25287427294368,0.9));
#24735=CARTESIAN_POINT('Ctrl Pts',(3.76001591476243,-1.34606837492147,0.9));
#24736=CARTESIAN_POINT('Ctrl Pts',(0.484117964332957,-1.06481006947648,
0.9));
#24737=CARTESIAN_POINT('Ctrl Pts',(10.3118118156214,-1.06114656258054,0.9));
#24738=CARTESIAN_POINT('Ctrl Pts',(10.3096972650911,-1.05897130198467,0.94150644476122));
#24739=CARTESIAN_POINT('Ctrl Pts',(10.3075827145608,-1.0567960413888,0.98301288952244));
#24740=CARTESIAN_POINT('Ctrl Pts',(10.3054681640305,-1.05462078079293,1.02451933428366));
#24741=CARTESIAN_POINT('Ctrl Pts',(7.03591386519191,-1.25287427294368,0.9));
#24742=CARTESIAN_POINT('Ctrl Pts',(7.03520959909601,-1.25069901234781,0.94150644476122));
#24743=CARTESIAN_POINT('Ctrl Pts',(7.03450533300011,-1.24852375175194,0.98301288952244));
#24744=CARTESIAN_POINT('Ctrl Pts',(7.03380106690421,-1.24634849115607,1.02451933428366));
#24745=CARTESIAN_POINT('Ctrl Pts',(3.76001591476244,-1.34606837492147,0.9));
#24746=CARTESIAN_POINT('Ctrl Pts',(3.76072193310095,-1.3438931143256,0.94150644476122));
#24747=CARTESIAN_POINT('Ctrl Pts',(3.76142795143946,-1.34171785372973,0.98301288952244));
#24748=CARTESIAN_POINT('Ctrl Pts',(3.76213396977796,-1.33954259313386,1.02451933428366));
#24749=CARTESIAN_POINT('Ctrl Pts',(0.484117964332957,-1.06481006947648,
0.9));
#24750=CARTESIAN_POINT('Ctrl Pts',(0.486234267105876,-1.06263480888061,
0.94150644476122));
#24751=CARTESIAN_POINT('Ctrl Pts',(0.488350569878795,-1.06045954828474,
0.98301288952244));
#24752=CARTESIAN_POINT('Ctrl Pts',(0.490466872651714,-1.05828428768887,
1.02451933428366));
#24794=UNCERTAINTY_MEASURE_WITH_UNIT(LENGTH_MEASURE(0.001),#24810,
'DISTANCE_ACCURACY_VALUE',
'Maximum model space distance between geometric entities at asserted c
onnectivities');
#24796=UNCERTAINTY_MEASURE_WITH_UNIT(LENGTH_MEASURE(0.001),#24810,
'DISTANCE_ACCURACY_VALUE',
'Maximum model space distance between geometric entities at asserted c
onnectivities');
#24807=(
GEOMETRIC_REPRESENTATION_CONTEXT(3)
GLOBAL_UNCERTAINTY_ASSIGNED_CONTEXT((#24794))
GLOBAL_UNIT_ASSIGNED_CONTEXT((#24810,#24812,#24813))
REPRESENTATION_CONTEXT('','3D')
);
#24809=(
GEOMETRIC_REPRESENTATION_CONTEXT(3)
GLOBAL_UNCERTAINTY_ASSIGNED_CONTEXT((#24796))
GLOBAL_UNIT_ASSIGNED_CONTEXT((#24810,#24812,#24813))
REPRESENTATION_CONTEXT('','3D')
);
#24810=(
LENGTH_UNIT()
NAMED_UNIT(*)
SI_UNIT(.CENTI.,.METRE.)
);
#24812=(
NAMED_UNIT(*)
PLANE_ANGLE_UNIT()
SI_UNIT($,.RADIAN.)
);
#24813=(
NAMED_UNIT(*)
SI_UNIT($,.STERADIAN.)
SOLID_ANGLE_UNIT()
);
#24824=SHAPE_DEFINITION_REPRESENTATION(#24836,#24864);
#24836=PRODUCT_DEFINITION_SHAPE('',$,#24877);
#24864=SHAPE_REPRESENTATION('',(#10595),#24807);
#24866=PRODUCT_DEFINITION_CONTEXT('part definition',#24904,'design');
#24877=PRODUCT_DEFINITION('2026-11-10-05-11-11-305','Soft grip layer',#24889,
#24866);
#24889=PRODUCT_DEFINITION_FORMATION('',$,#24916);
#24904=APPLICATION_CONTEXT(
'Core Data for Automotive Mechanical Design Process');
#24905=PRODUCT_CONTEXT('part definition',#24904,'mechanical');
#24916=PRODUCT('2026-11-10-05-11-11-305','Soft grip layer',$,(#24905));
#24924=PRESENTATION_STYLE_ASSIGNMENT((#24932));
#24932=SURFACE_STYLE_USAGE(.BOTH.,#24940);
#24940=SURFACE_SIDE_STYLE('',(#24948));
#24948=SURFACE_STYLE_FILL_AREA(#24956);
#24956=FILL_AREA_STYLE('Sky blue soft grip',(#24964));
#24964=FILL_AREA_STYLE_COLOUR('Sky blue soft grip',#24972);
#24972=COLOUR_RGB('Sky blue soft grip',0.317647058823529,0.686274509803922,
0.890196078431372);
ENDSEC;
END-ISO-10303-21;
